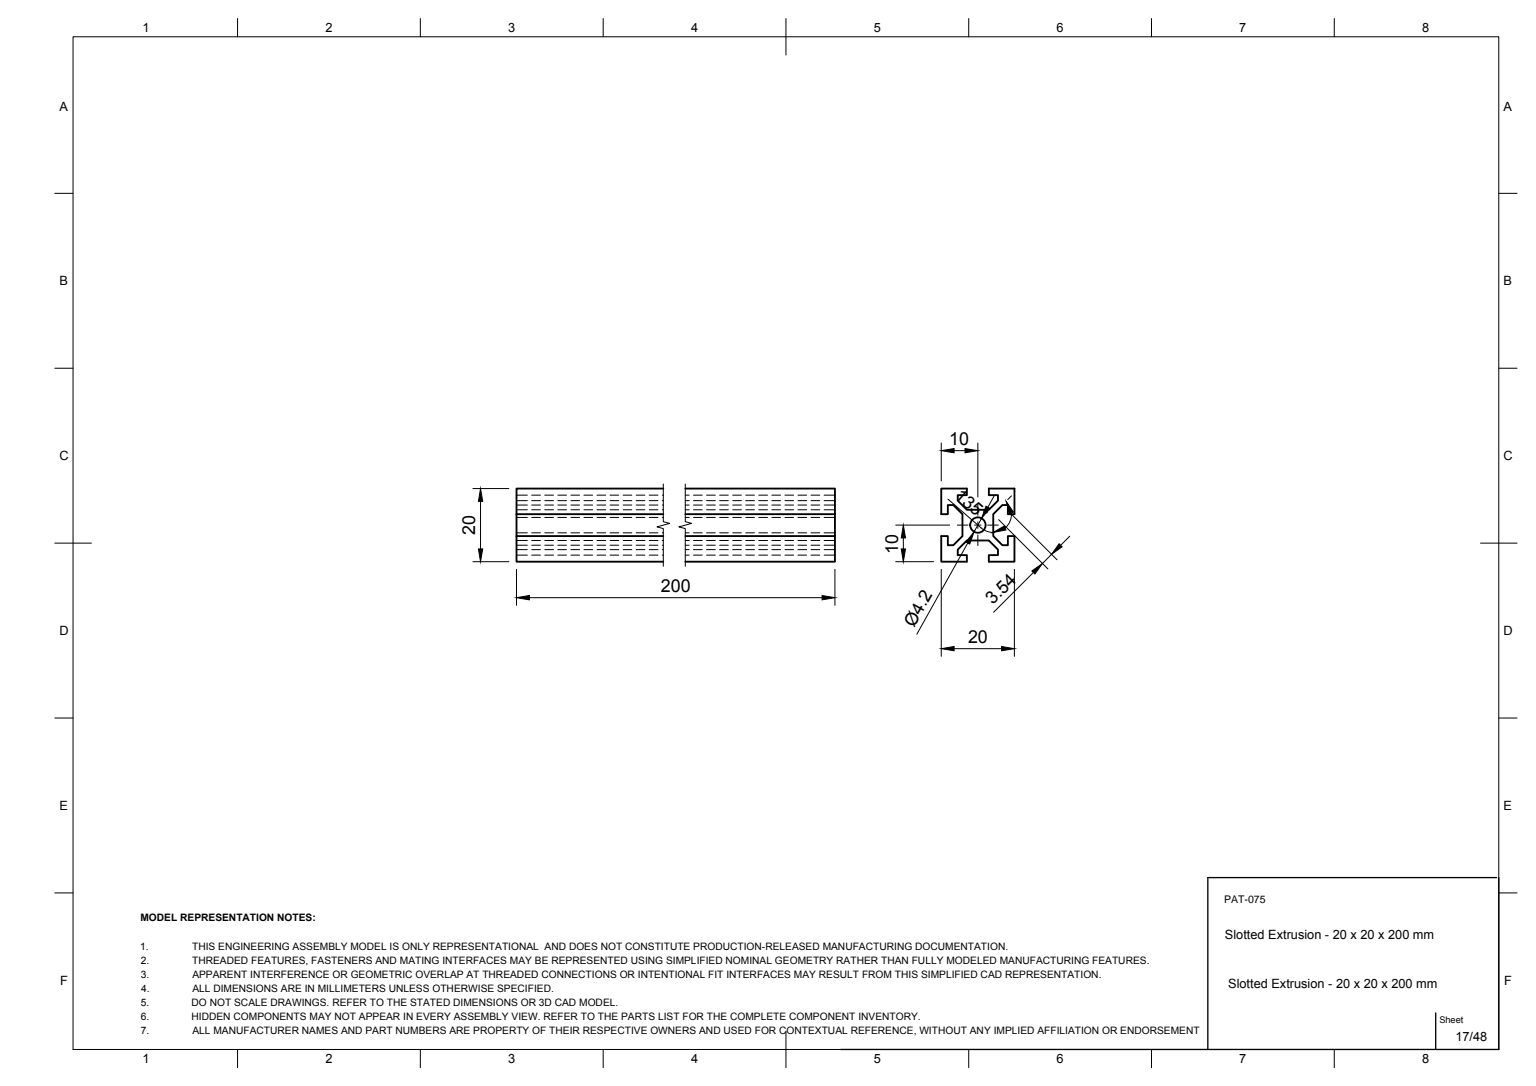
ISO-10303-21;
HEADER;
/* Generated by software containing ST-Developer
 * from STEP Tools, Inc. (www.steptools.com) 
 */

FILE_DESCRIPTION(
/* description */ ('Over-Centre Plunger Toggle Clamp on Slotted Fixture Frame'),
/* implementation_level */ '2;1');

FILE_NAME(
/* name */ 
'Slotted Extrusion - 20 x 20 x 200 mm.step',
/* time_stamp */ '2026-10-28T03:23:24-07:00',
/* author */ (''),
/* organization */ (''),
/* preprocessor_version */ 'ST-DEVELOPER v20.2',
/* originating_system */ 'Autodesk Translation Framework v15.17.0.0',
/* authorisation */ '');

FILE_SCHEMA (('AUTOMOTIVE_DESIGN { 1 0 10303 214 3 1 1 }'));
ENDSEC;

DATA;
#10=MECHANICAL_DESIGN_GEOMETRIC_PRESENTATION_REPRESENTATION('',(#525),#15212);
#441=SHAPE_REPRESENTATION_RELATIONSHIP('SRR','None',#15415,#483);
#483=ADVANCED_BREP_SHAPE_REPRESENTATION('',(#576),#15177);
#525=STYLED_ITEM('',(#15733),#576);
#576=MANIFOLD_SOLID_BREP('Body1',#8257);
#714=FACE_BOUND('',#1871,.T.);
#715=FACE_BOUND('',#1873,.T.);
#866=PLANE('',#9059);
#867=PLANE('',#9060);
#868=PLANE('',#9061);
#869=PLANE('',#9062);
#870=PLANE('',#9063);
#871=PLANE('',#9064);
#872=PLANE('',#9065);
#873=PLANE('',#9066);
#874=PLANE('',#9067);
#875=PLANE('',#9068);
#876=PLANE('',#9069);
#877=PLANE('',#9070);
#878=PLANE('',#9071);
#879=PLANE('',#9072);
#880=PLANE('',#9073);
#881=PLANE('',#9074);
#882=PLANE('',#9075);
#883=PLANE('',#9076);
#884=PLANE('',#9077);
#885=PLANE('',#9078);
#886=PLANE('',#9079);
#887=PLANE('',#9080);
#888=PLANE('',#9081);
#889=PLANE('',#9082);
#890=PLANE('',#9083);
#891=PLANE('',#9084);
#892=PLANE('',#9085);
#893=PLANE('',#9086);
#894=PLANE('',#9087);
#895=PLANE('',#9088);
#896=PLANE('',#9089);
#897=PLANE('',#9090);
#898=PLANE('',#9091);
#899=PLANE('',#9092);
#900=PLANE('',#9093);
#901=PLANE('',#9094);
#902=PLANE('',#9098);
#903=PLANE('',#9099);
#904=PLANE('',#9100);
#905=PLANE('',#9101);
#906=PLANE('',#9102);
#907=PLANE('',#9103);
#908=PLANE('',#9104);
#909=PLANE('',#9105);
#910=PLANE('',#9106);
#911=PLANE('',#9107);
#1236=FACE_OUTER_BOUND('',#1825,.T.);
#1237=FACE_OUTER_BOUND('',#1826,.T.);
#1238=FACE_OUTER_BOUND('',#1827,.T.);
#1239=FACE_OUTER_BOUND('',#1828,.T.);
#1240=FACE_OUTER_BOUND('',#1829,.T.);
#1241=FACE_OUTER_BOUND('',#1830,.T.);
#1242=FACE_OUTER_BOUND('',#1831,.T.);
#1243=FACE_OUTER_BOUND('',#1832,.T.);
#1244=FACE_OUTER_BOUND('',#1833,.T.);
#1245=FACE_OUTER_BOUND('',#1834,.T.);
#1246=FACE_OUTER_BOUND('',#1835,.T.);
#1247=FACE_OUTER_BOUND('',#1836,.T.);
#1248=FACE_OUTER_BOUND('',#1837,.T.);
#1249=FACE_OUTER_BOUND('',#1838,.T.);
#1250=FACE_OUTER_BOUND('',#1839,.T.);
#1251=FACE_OUTER_BOUND('',#1840,.T.);
#1252=FACE_OUTER_BOUND('',#1841,.T.);
#1253=FACE_OUTER_BOUND('',#1842,.T.);
#1254=FACE_OUTER_BOUND('',#1843,.T.);
#1255=FACE_OUTER_BOUND('',#1844,.T.);
#1256=FACE_OUTER_BOUND('',#1845,.T.);
#1257=FACE_OUTER_BOUND('',#1846,.T.);
#1258=FACE_OUTER_BOUND('',#1847,.T.);
#1259=FACE_OUTER_BOUND('',#1848,.T.);
#1260=FACE_OUTER_BOUND('',#1849,.T.);
#1261=FACE_OUTER_BOUND('',#1850,.T.);
#1262=FACE_OUTER_BOUND('',#1851,.T.);
#1263=FACE_OUTER_BOUND('',#1852,.T.);
#1264=FACE_OUTER_BOUND('',#1853,.T.);
#1265=FACE_OUTER_BOUND('',#1854,.T.);
#1266=FACE_OUTER_BOUND('',#1855,.T.);
#1267=FACE_OUTER_BOUND('',#1856,.T.);
#1268=FACE_OUTER_BOUND('',#1857,.T.);
#1269=FACE_OUTER_BOUND('',#1858,.T.);
#1270=FACE_OUTER_BOUND('',#1859,.T.);
#1271=FACE_OUTER_BOUND('',#1860,.T.);
#1272=FACE_OUTER_BOUND('',#1861,.T.);
#1273=FACE_OUTER_BOUND('',#1862,.T.);
#1274=FACE_OUTER_BOUND('',#1863,.T.);
#1275=FACE_OUTER_BOUND('',#1864,.T.);
#1276=FACE_OUTER_BOUND('',#1865,.T.);
#1277=FACE_OUTER_BOUND('',#1866,.T.);
#1278=FACE_OUTER_BOUND('',#1867,.T.);
#1279=FACE_OUTER_BOUND('',#1868,.T.);
#1280=FACE_OUTER_BOUND('',#1869,.T.);
#1281=FACE_OUTER_BOUND('',#1870,.T.);
#1282=FACE_OUTER_BOUND('',#1872,.T.);
#1825=EDGE_LOOP('',(#6205,#6206,#6207,#6208));
#1826=EDGE_LOOP('',(#6209,#6210,#6211,#6212));
#1827=EDGE_LOOP('',(#6213,#6214,#6215,#6216));
#1828=EDGE_LOOP('',(#6217,#6218,#6219,#6220));
#1829=EDGE_LOOP('',(#6221,#6222,#6223,#6224));
#1830=EDGE_LOOP('',(#6225,#6226,#6227,#6228));
#1831=EDGE_LOOP('',(#6229,#6230,#6231,#6232));
#1832=EDGE_LOOP('',(#6233,#6234,#6235,#6236));
#1833=EDGE_LOOP('',(#6237,#6238,#6239,#6240));
#1834=EDGE_LOOP('',(#6241,#6242,#6243,#6244));
#1835=EDGE_LOOP('',(#6245,#6246,#6247,#6248));
#1836=EDGE_LOOP('',(#6249,#6250,#6251,#6252));
#1837=EDGE_LOOP('',(#6253,#6254,#6255,#6256));
#1838=EDGE_LOOP('',(#6257,#6258,#6259,#6260));
#1839=EDGE_LOOP('',(#6261,#6262,#6263,#6264));
#1840=EDGE_LOOP('',(#6265,#6266,#6267,#6268));
#1841=EDGE_LOOP('',(#6269,#6270,#6271,#6272));
#1842=EDGE_LOOP('',(#6273,#6274,#6275,#6276));
#1843=EDGE_LOOP('',(#6277,#6278,#6279,#6280));
#1844=EDGE_LOOP('',(#6281,#6282,#6283,#6284));
#1845=EDGE_LOOP('',(#6285,#6286,#6287,#6288));
#1846=EDGE_LOOP('',(#6289,#6290,#6291,#6292));
#1847=EDGE_LOOP('',(#6293,#6294,#6295,#6296));
#1848=EDGE_LOOP('',(#6297,#6298,#6299,#6300));
#1849=EDGE_LOOP('',(#6301,#6302,#6303,#6304));
#1850=EDGE_LOOP('',(#6305,#6306,#6307,#6308));
#1851=EDGE_LOOP('',(#6309,#6310,#6311,#6312));
#1852=EDGE_LOOP('',(#6313,#6314,#6315,#6316));
#1853=EDGE_LOOP('',(#6317,#6318,#6319,#6320));
#1854=EDGE_LOOP('',(#6321,#6322,#6323,#6324));
#1855=EDGE_LOOP('',(#6325,#6326,#6327,#6328));
#1856=EDGE_LOOP('',(#6329,#6330,#6331,#6332));
#1857=EDGE_LOOP('',(#6333,#6334,#6335,#6336));
#1858=EDGE_LOOP('',(#6337,#6338,#6339,#6340));
#1859=EDGE_LOOP('',(#6341,#6342,#6343,#6344));
#1860=EDGE_LOOP('',(#6345,#6346,#6347,#6348));
#1861=EDGE_LOOP('',(#6349,#6350,#6351,#6352));
#1862=EDGE_LOOP('',(#6353,#6354,#6355,#6356));
#1863=EDGE_LOOP('',(#6357,#6358,#6359,#6360));
#1864=EDGE_LOOP('',(#6361,#6362,#6363,#6364));
#1865=EDGE_LOOP('',(#6365,#6366,#6367,#6368));
#1866=EDGE_LOOP('',(#6369,#6370,#6371,#6372));
#1867=EDGE_LOOP('',(#6373,#6374,#6375,#6376));
#1868=EDGE_LOOP('',(#6377,#6378,#6379,#6380));
#1869=EDGE_LOOP('',(#6381,#6382,#6383,#6384));
#1870=EDGE_LOOP('',(#6385,#6386,#6387,#6388,#6389,#6390,#6391,#6392,#6393,
#6394,#6395,#6396,#6397,#6398,#6399,#6400,#6401,#6402,#6403,#6404,#6405,
#6406,#6407,#6408,#6409,#6410,#6411,#6412,#6413,#6414,#6415,#6416,#6417,
#6418,#6419,#6420,#6421,#6422,#6423,#6424,#6425,#6426,#6427,#6428));
#1871=EDGE_LOOP('',(#6429));
#1872=EDGE_LOOP('',(#6430,#6431,#6432,#6433,#6434,#6435,#6436,#6437,#6438,
#6439,#6440,#6441,#6442,#6443,#6444,#6445,#6446,#6447,#6448,#6449,#6450,
#6451,#6452,#6453,#6454,#6455,#6456,#6457,#6458,#6459,#6460,#6461,#6462,
#6463,#6464,#6465,#6466,#6467,#6468,#6469,#6470,#6471,#6472,#6473));
#1873=EDGE_LOOP('',(#6474));
#2417=LINE('',#13063,#3047);
#2418=LINE('',#13065,#3048);
#2419=LINE('',#13067,#3049);
#2420=LINE('',#13068,#3050);
#2421=LINE('',#13071,#3051);
#2422=LINE('',#13073,#3052);
#2423=LINE('',#13074,#3053);
#2424=LINE('',#13077,#3054);
#2425=LINE('',#13079,#3055);
#2426=LINE('',#13080,#3056);
#2427=LINE('',#13083,#3057);
#2428=LINE('',#13085,#3058);
#2429=LINE('',#13086,#3059);
#2430=LINE('',#13089,#3060);
#2431=LINE('',#13091,#3061);
#2432=LINE('',#13092,#3062);
#2433=LINE('',#13095,#3063);
#2434=LINE('',#13097,#3064);
#2435=LINE('',#13098,#3065);
#2436=LINE('',#13101,#3066);
#2437=LINE('',#13103,#3067);
#2438=LINE('',#13104,#3068);
#2439=LINE('',#13107,#3069);
#2440=LINE('',#13109,#3070);
#2441=LINE('',#13110,#3071);
#2442=LINE('',#13113,#3072);
#2443=LINE('',#13115,#3073);
#2444=LINE('',#13116,#3074);
#2445=LINE('',#13120,#3075);
#2446=LINE('',#13122,#3076);
#2447=LINE('',#13124,#3077);
#2448=LINE('',#13125,#3078);
#2449=LINE('',#13128,#3079);
#2450=LINE('',#13130,#3080);
#2451=LINE('',#13131,#3081);
#2452=LINE('',#13134,#3082);
#2453=LINE('',#13136,#3083);
#2454=LINE('',#13137,#3084);
#2455=LINE('',#13140,#3085);
#2456=LINE('',#13142,#3086);
#2457=LINE('',#13143,#3087);
#2458=LINE('',#13146,#3088);
#2459=LINE('',#13148,#3089);
#2460=LINE('',#13149,#3090);
#2461=LINE('',#13152,#3091);
#2462=LINE('',#13154,#3092);
#2463=LINE('',#13155,#3093);
#2464=LINE('',#13158,#3094);
#2465=LINE('',#13160,#3095);
#2466=LINE('',#13161,#3096);
#2467=LINE('',#13164,#3097);
#2468=LINE('',#13166,#3098);
#2469=LINE('',#13167,#3099);
#2470=LINE('',#13170,#3100);
#2471=LINE('',#13172,#3101);
#2472=LINE('',#13173,#3102);
#2473=LINE('',#13177,#3103);
#2474=LINE('',#13179,#3104);
#2475=LINE('',#13181,#3105);
#2476=LINE('',#13182,#3106);
#2477=LINE('',#13185,#3107);
#2478=LINE('',#13187,#3108);
#2479=LINE('',#13188,#3109);
#2480=LINE('',#13191,#3110);
#2481=LINE('',#13193,#3111);
#2482=LINE('',#13194,#3112);
#2483=LINE('',#13197,#3113);
#2484=LINE('',#13199,#3114);
#2485=LINE('',#13200,#3115);
#2486=LINE('',#13203,#3116);
#2487=LINE('',#13205,#3117);
#2488=LINE('',#13206,#3118);
#2489=LINE('',#13209,#3119);
#2490=LINE('',#13211,#3120);
#2491=LINE('',#13212,#3121);
#2492=LINE('',#13215,#3122);
#2493=LINE('',#13217,#3123);
#2494=LINE('',#13218,#3124);
#2495=LINE('',#13221,#3125);
#2496=LINE('',#13223,#3126);
#2497=LINE('',#13224,#3127);
#2498=LINE('',#13227,#3128);
#2499=LINE('',#13229,#3129);
#2500=LINE('',#13230,#3130);
#2501=LINE('',#13234,#3131);
#2502=LINE('',#13236,#3132);
#2503=LINE('',#13238,#3133);
#2504=LINE('',#13239,#3134);
#2505=LINE('',#13242,#3135);
#2506=LINE('',#13244,#3136);
#2507=LINE('',#13245,#3137);
#2508=LINE('',#13248,#3138);
#2509=LINE('',#13250,#3139);
#2510=LINE('',#13251,#3140);
#2511=LINE('',#13254,#3141);
#2512=LINE('',#13256,#3142);
#2513=LINE('',#13257,#3143);
#2514=LINE('',#13260,#3144);
#2515=LINE('',#13262,#3145);
#2516=LINE('',#13263,#3146);
#2517=LINE('',#13266,#3147);
#2518=LINE('',#13268,#3148);
#2519=LINE('',#13269,#3149);
#2520=LINE('',#13272,#3150);
#2521=LINE('',#13274,#3151);
#2522=LINE('',#13275,#3152);
#2523=LINE('',#13278,#3153);
#2524=LINE('',#13280,#3154);
#2525=LINE('',#13281,#3155);
#2526=LINE('',#13284,#3156);
#2527=LINE('',#13286,#3157);
#2528=LINE('',#13287,#3158);
#2529=LINE('',#13292,#3159);
#2530=LINE('',#13296,#3160);
#2531=LINE('',#13298,#3161);
#2532=LINE('',#13299,#3162);
#2533=LINE('',#13302,#3163);
#2534=LINE('',#13304,#3164);
#2535=LINE('',#13305,#3165);
#2536=LINE('',#13307,#3166);
#2537=LINE('',#13308,#3167);
#2538=LINE('',#13311,#3168);
#2539=LINE('',#13313,#3169);
#2540=LINE('',#13314,#3170);
#2541=LINE('',#13316,#3171);
#2542=LINE('',#13317,#3172);
#2543=LINE('',#13320,#3173);
#2544=LINE('',#13322,#3174);
#2545=LINE('',#13323,#3175);
#2546=LINE('',#13325,#3176);
#2547=LINE('',#13326,#3177);
#2548=LINE('',#13328,#3178);
#2549=LINE('',#13329,#3179);
#3047=VECTOR('',#10534,1.);
#3048=VECTOR('',#10535,1.);
#3049=VECTOR('',#10536,1.);
#3050=VECTOR('',#10537,1.);
#3051=VECTOR('',#10540,1.);
#3052=VECTOR('',#10541,1.);
#3053=VECTOR('',#10542,1.);
#3054=VECTOR('',#10545,1.);
#3055=VECTOR('',#10546,1.);
#3056=VECTOR('',#10547,1.);
#3057=VECTOR('',#10550,1.);
#3058=VECTOR('',#10551,1.);
#3059=VECTOR('',#10552,1.);
#3060=VECTOR('',#10555,1.);
#3061=VECTOR('',#10556,1.);
#3062=VECTOR('',#10557,1.);
#3063=VECTOR('',#10560,1.);
#3064=VECTOR('',#10561,1.);
#3065=VECTOR('',#10562,1.);
#3066=VECTOR('',#10565,1.);
#3067=VECTOR('',#10566,1.);
#3068=VECTOR('',#10567,1.);
#3069=VECTOR('',#10570,1.);
#3070=VECTOR('',#10571,1.);
#3071=VECTOR('',#10572,1.);
#3072=VECTOR('',#10575,1.);
#3073=VECTOR('',#10576,1.);
#3074=VECTOR('',#10577,1.);
#3075=VECTOR('',#10580,1.);
#3076=VECTOR('',#10581,1.);
#3077=VECTOR('',#10582,1.);
#3078=VECTOR('',#10583,1.);
#3079=VECTOR('',#10586,1.);
#3080=VECTOR('',#10587,1.);
#3081=VECTOR('',#10588,1.);
#3082=VECTOR('',#10591,1.);
#3083=VECTOR('',#10592,1.);
#3084=VECTOR('',#10593,1.);
#3085=VECTOR('',#10596,1.);
#3086=VECTOR('',#10597,1.);
#3087=VECTOR('',#10598,1.);
#3088=VECTOR('',#10601,1.);
#3089=VECTOR('',#10602,1.);
#3090=VECTOR('',#10603,1.);
#3091=VECTOR('',#10606,1.);
#3092=VECTOR('',#10607,1.);
#3093=VECTOR('',#10608,1.);
#3094=VECTOR('',#10611,1.);
#3095=VECTOR('',#10612,1.);
#3096=VECTOR('',#10613,1.);
#3097=VECTOR('',#10616,1.);
#3098=VECTOR('',#10617,1.);
#3099=VECTOR('',#10618,1.);
#3100=VECTOR('',#10621,1.);
#3101=VECTOR('',#10622,1.);
#3102=VECTOR('',#10623,1.);
#3103=VECTOR('',#10626,1.);
#3104=VECTOR('',#10627,1.);
#3105=VECTOR('',#10628,1.);
#3106=VECTOR('',#10629,1.);
#3107=VECTOR('',#10632,1.);
#3108=VECTOR('',#10633,1.);
#3109=VECTOR('',#10634,1.);
#3110=VECTOR('',#10637,1.);
#3111=VECTOR('',#10638,1.);
#3112=VECTOR('',#10639,1.);
#3113=VECTOR('',#10642,1.);
#3114=VECTOR('',#10643,1.);
#3115=VECTOR('',#10644,1.);
#3116=VECTOR('',#10647,1.);
#3117=VECTOR('',#10648,1.);
#3118=VECTOR('',#10649,1.);
#3119=VECTOR('',#10652,1.);
#3120=VECTOR('',#10653,1.);
#3121=VECTOR('',#10654,1.);
#3122=VECTOR('',#10657,1.);
#3123=VECTOR('',#10658,1.);
#3124=VECTOR('',#10659,1.);
#3125=VECTOR('',#10662,1.);
#3126=VECTOR('',#10663,1.);
#3127=VECTOR('',#10664,1.);
#3128=VECTOR('',#10667,1.);
#3129=VECTOR('',#10668,1.);
#3130=VECTOR('',#10669,1.);
#3131=VECTOR('',#10672,1.);
#3132=VECTOR('',#10673,1.);
#3133=VECTOR('',#10674,1.);
#3134=VECTOR('',#10675,1.);
#3135=VECTOR('',#10678,1.);
#3136=VECTOR('',#10679,1.);
#3137=VECTOR('',#10680,1.);
#3138=VECTOR('',#10683,1.);
#3139=VECTOR('',#10684,1.);
#3140=VECTOR('',#10685,1.);
#3141=VECTOR('',#10688,1.);
#3142=VECTOR('',#10689,1.);
#3143=VECTOR('',#10690,1.);
#3144=VECTOR('',#10693,1.);
#3145=VECTOR('',#10694,1.);
#3146=VECTOR('',#10695,1.);
#3147=VECTOR('',#10698,1.);
#3148=VECTOR('',#10699,1.);
#3149=VECTOR('',#10700,1.);
#3150=VECTOR('',#10703,1.);
#3151=VECTOR('',#10704,1.);
#3152=VECTOR('',#10705,1.);
#3153=VECTOR('',#10708,1.);
#3154=VECTOR('',#10709,1.);
#3155=VECTOR('',#10710,1.);
#3156=VECTOR('',#10713,1.);
#3157=VECTOR('',#10714,1.);
#3158=VECTOR('',#10715,1.);
#3159=VECTOR('',#10720,0.21);
#3160=VECTOR('',#10725,1.);
#3161=VECTOR('',#10726,1.);
#3162=VECTOR('',#10727,1.);
#3163=VECTOR('',#10730,1.);
#3164=VECTOR('',#10731,1.);
#3165=VECTOR('',#10732,1.);
#3166=VECTOR('',#10735,1.);
#3167=VECTOR('',#10736,1.);
#3168=VECTOR('',#10739,1.);
#3169=VECTOR('',#10740,1.);
#3170=VECTOR('',#10741,1.);
#3171=VECTOR('',#10744,1.);
#3172=VECTOR('',#10745,1.);
#3173=VECTOR('',#10748,1.);
#3174=VECTOR('',#10749,1.);
#3175=VECTOR('',#10750,1.);
#3176=VECTOR('',#10753,1.);
#3177=VECTOR('',#10754,1.);
#3178=VECTOR('',#10757,1.);
#3179=VECTOR('',#10758,1.);
#3623=CIRCLE('',#9096,0.21);
#3624=CIRCLE('',#9097,0.21);
#4071=VERTEX_POINT('',#13061);
#4072=VERTEX_POINT('',#13062);
#4073=VERTEX_POINT('',#13064);
#4074=VERTEX_POINT('',#13066);
#4075=VERTEX_POINT('',#13070);
#4076=VERTEX_POINT('',#13072);
#4077=VERTEX_POINT('',#13076);
#4078=VERTEX_POINT('',#13078);
#4079=VERTEX_POINT('',#13082);
#4080=VERTEX_POINT('',#13084);
#4081=VERTEX_POINT('',#13088);
#4082=VERTEX_POINT('',#13090);
#4083=VERTEX_POINT('',#13094);
#4084=VERTEX_POINT('',#13096);
#4085=VERTEX_POINT('',#13100);
#4086=VERTEX_POINT('',#13102);
#4087=VERTEX_POINT('',#13106);
#4088=VERTEX_POINT('',#13108);
#4089=VERTEX_POINT('',#13112);
#4090=VERTEX_POINT('',#13114);
#4091=VERTEX_POINT('',#13118);
#4092=VERTEX_POINT('',#13119);
#4093=VERTEX_POINT('',#13121);
#4094=VERTEX_POINT('',#13123);
#4095=VERTEX_POINT('',#13127);
#4096=VERTEX_POINT('',#13129);
#4097=VERTEX_POINT('',#13133);
#4098=VERTEX_POINT('',#13135);
#4099=VERTEX_POINT('',#13139);
#4100=VERTEX_POINT('',#13141);
#4101=VERTEX_POINT('',#13145);
#4102=VERTEX_POINT('',#13147);
#4103=VERTEX_POINT('',#13151);
#4104=VERTEX_POINT('',#13153);
#4105=VERTEX_POINT('',#13157);
#4106=VERTEX_POINT('',#13159);
#4107=VERTEX_POINT('',#13163);
#4108=VERTEX_POINT('',#13165);
#4109=VERTEX_POINT('',#13169);
#4110=VERTEX_POINT('',#13171);
#4111=VERTEX_POINT('',#13175);
#4112=VERTEX_POINT('',#13176);
#4113=VERTEX_POINT('',#13178);
#4114=VERTEX_POINT('',#13180);
#4115=VERTEX_POINT('',#13184);
#4116=VERTEX_POINT('',#13186);
#4117=VERTEX_POINT('',#13190);
#4118=VERTEX_POINT('',#13192);
#4119=VERTEX_POINT('',#13196);
#4120=VERTEX_POINT('',#13198);
#4121=VERTEX_POINT('',#13202);
#4122=VERTEX_POINT('',#13204);
#4123=VERTEX_POINT('',#13208);
#4124=VERTEX_POINT('',#13210);
#4125=VERTEX_POINT('',#13214);
#4126=VERTEX_POINT('',#13216);
#4127=VERTEX_POINT('',#13220);
#4128=VERTEX_POINT('',#13222);
#4129=VERTEX_POINT('',#13226);
#4130=VERTEX_POINT('',#13228);
#4131=VERTEX_POINT('',#13232);
#4132=VERTEX_POINT('',#13233);
#4133=VERTEX_POINT('',#13235);
#4134=VERTEX_POINT('',#13237);
#4135=VERTEX_POINT('',#13241);
#4136=VERTEX_POINT('',#13243);
#4137=VERTEX_POINT('',#13247);
#4138=VERTEX_POINT('',#13249);
#4139=VERTEX_POINT('',#13253);
#4140=VERTEX_POINT('',#13255);
#4141=VERTEX_POINT('',#13259);
#4142=VERTEX_POINT('',#13261);
#4143=VERTEX_POINT('',#13265);
#4144=VERTEX_POINT('',#13267);
#4145=VERTEX_POINT('',#13271);
#4146=VERTEX_POINT('',#13273);
#4147=VERTEX_POINT('',#13277);
#4148=VERTEX_POINT('',#13279);
#4149=VERTEX_POINT('',#13283);
#4150=VERTEX_POINT('',#13285);
#4151=VERTEX_POINT('',#13289);
#4152=VERTEX_POINT('',#13291);
#4153=VERTEX_POINT('',#13295);
#4154=VERTEX_POINT('',#13297);
#4155=VERTEX_POINT('',#13301);
#4156=VERTEX_POINT('',#13303);
#4157=VERTEX_POINT('',#13310);
#4158=VERTEX_POINT('',#13312);
#4159=VERTEX_POINT('',#13319);
#4160=VERTEX_POINT('',#13321);
#4863=EDGE_CURVE('',#4071,#4072,#2417,.T.);
#4864=EDGE_CURVE('',#4071,#4073,#2418,.T.);
#4865=EDGE_CURVE('',#4074,#4073,#2419,.T.);
#4866=EDGE_CURVE('',#4072,#4074,#2420,.T.);
#4867=EDGE_CURVE('',#4075,#4071,#2421,.T.);
#4868=EDGE_CURVE('',#4075,#4076,#2422,.T.);
#4869=EDGE_CURVE('',#4073,#4076,#2423,.T.);
#4870=EDGE_CURVE('',#4077,#4075,#2424,.T.);
#4871=EDGE_CURVE('',#4077,#4078,#2425,.T.);
#4872=EDGE_CURVE('',#4076,#4078,#2426,.T.);
#4873=EDGE_CURVE('',#4079,#4077,#2427,.T.);
#4874=EDGE_CURVE('',#4079,#4080,#2428,.T.);
#4875=EDGE_CURVE('',#4078,#4080,#2429,.T.);
#4876=EDGE_CURVE('',#4081,#4079,#2430,.T.);
#4877=EDGE_CURVE('',#4081,#4082,#2431,.T.);
#4878=EDGE_CURVE('',#4080,#4082,#2432,.T.);
#4879=EDGE_CURVE('',#4083,#4081,#2433,.T.);
#4880=EDGE_CURVE('',#4083,#4084,#2434,.T.);
#4881=EDGE_CURVE('',#4082,#4084,#2435,.T.);
#4882=EDGE_CURVE('',#4085,#4083,#2436,.T.);
#4883=EDGE_CURVE('',#4085,#4086,#2437,.T.);
#4884=EDGE_CURVE('',#4084,#4086,#2438,.T.);
#4885=EDGE_CURVE('',#4087,#4085,#2439,.T.);
#4886=EDGE_CURVE('',#4087,#4088,#2440,.T.);
#4887=EDGE_CURVE('',#4086,#4088,#2441,.T.);
#4888=EDGE_CURVE('',#4089,#4087,#2442,.T.);
#4889=EDGE_CURVE('',#4090,#4089,#2443,.T.);
#4890=EDGE_CURVE('',#4088,#4090,#2444,.T.);
#4891=EDGE_CURVE('',#4091,#4092,#2445,.T.);
#4892=EDGE_CURVE('',#4091,#4093,#2446,.T.);
#4893=EDGE_CURVE('',#4094,#4093,#2447,.T.);
#4894=EDGE_CURVE('',#4092,#4094,#2448,.T.);
#4895=EDGE_CURVE('',#4095,#4091,#2449,.T.);
#4896=EDGE_CURVE('',#4095,#4096,#2450,.T.);
#4897=EDGE_CURVE('',#4093,#4096,#2451,.T.);
#4898=EDGE_CURVE('',#4097,#4095,#2452,.T.);
#4899=EDGE_CURVE('',#4097,#4098,#2453,.T.);
#4900=EDGE_CURVE('',#4096,#4098,#2454,.T.);
#4901=EDGE_CURVE('',#4099,#4097,#2455,.T.);
#4902=EDGE_CURVE('',#4099,#4100,#2456,.T.);
#4903=EDGE_CURVE('',#4098,#4100,#2457,.T.);
#4904=EDGE_CURVE('',#4101,#4099,#2458,.T.);
#4905=EDGE_CURVE('',#4101,#4102,#2459,.T.);
#4906=EDGE_CURVE('',#4100,#4102,#2460,.T.);
#4907=EDGE_CURVE('',#4103,#4101,#2461,.T.);
#4908=EDGE_CURVE('',#4103,#4104,#2462,.T.);
#4909=EDGE_CURVE('',#4102,#4104,#2463,.T.);
#4910=EDGE_CURVE('',#4105,#4103,#2464,.T.);
#4911=EDGE_CURVE('',#4105,#4106,#2465,.T.);
#4912=EDGE_CURVE('',#4104,#4106,#2466,.T.);
#4913=EDGE_CURVE('',#4107,#4105,#2467,.T.);
#4914=EDGE_CURVE('',#4107,#4108,#2468,.T.);
#4915=EDGE_CURVE('',#4106,#4108,#2469,.T.);
#4916=EDGE_CURVE('',#4109,#4107,#2470,.T.);
#4917=EDGE_CURVE('',#4110,#4109,#2471,.T.);
#4918=EDGE_CURVE('',#4108,#4110,#2472,.T.);
#4919=EDGE_CURVE('',#4111,#4112,#2473,.T.);
#4920=EDGE_CURVE('',#4111,#4113,#2474,.T.);
#4921=EDGE_CURVE('',#4114,#4113,#2475,.T.);
#4922=EDGE_CURVE('',#4112,#4114,#2476,.T.);
#4923=EDGE_CURVE('',#4115,#4111,#2477,.T.);
#4924=EDGE_CURVE('',#4115,#4116,#2478,.T.);
#4925=EDGE_CURVE('',#4113,#4116,#2479,.T.);
#4926=EDGE_CURVE('',#4117,#4115,#2480,.T.);
#4927=EDGE_CURVE('',#4117,#4118,#2481,.T.);
#4928=EDGE_CURVE('',#4116,#4118,#2482,.T.);
#4929=EDGE_CURVE('',#4119,#4117,#2483,.T.);
#4930=EDGE_CURVE('',#4119,#4120,#2484,.T.);
#4931=EDGE_CURVE('',#4118,#4120,#2485,.T.);
#4932=EDGE_CURVE('',#4121,#4119,#2486,.T.);
#4933=EDGE_CURVE('',#4121,#4122,#2487,.T.);
#4934=EDGE_CURVE('',#4120,#4122,#2488,.T.);
#4935=EDGE_CURVE('',#4123,#4121,#2489,.T.);
#4936=EDGE_CURVE('',#4123,#4124,#2490,.T.);
#4937=EDGE_CURVE('',#4122,#4124,#2491,.T.);
#4938=EDGE_CURVE('',#4125,#4123,#2492,.T.);
#4939=EDGE_CURVE('',#4125,#4126,#2493,.T.);
#4940=EDGE_CURVE('',#4124,#4126,#2494,.T.);
#4941=EDGE_CURVE('',#4127,#4125,#2495,.T.);
#4942=EDGE_CURVE('',#4127,#4128,#2496,.T.);
#4943=EDGE_CURVE('',#4126,#4128,#2497,.T.);
#4944=EDGE_CURVE('',#4129,#4127,#2498,.T.);
#4945=EDGE_CURVE('',#4130,#4129,#2499,.T.);
#4946=EDGE_CURVE('',#4128,#4130,#2500,.T.);
#4947=EDGE_CURVE('',#4131,#4132,#2501,.T.);
#4948=EDGE_CURVE('',#4131,#4133,#2502,.T.);
#4949=EDGE_CURVE('',#4134,#4133,#2503,.T.);
#4950=EDGE_CURVE('',#4132,#4134,#2504,.T.);
#4951=EDGE_CURVE('',#4135,#4131,#2505,.T.);
#4952=EDGE_CURVE('',#4135,#4136,#2506,.T.);
#4953=EDGE_CURVE('',#4133,#4136,#2507,.T.);
#4954=EDGE_CURVE('',#4137,#4135,#2508,.T.);
#4955=EDGE_CURVE('',#4137,#4138,#2509,.T.);
#4956=EDGE_CURVE('',#4136,#4138,#2510,.T.);
#4957=EDGE_CURVE('',#4139,#4137,#2511,.T.);
#4958=EDGE_CURVE('',#4139,#4140,#2512,.T.);
#4959=EDGE_CURVE('',#4138,#4140,#2513,.T.);
#4960=EDGE_CURVE('',#4141,#4139,#2514,.T.);
#4961=EDGE_CURVE('',#4141,#4142,#2515,.T.);
#4962=EDGE_CURVE('',#4140,#4142,#2516,.T.);
#4963=EDGE_CURVE('',#4143,#4141,#2517,.T.);
#4964=EDGE_CURVE('',#4143,#4144,#2518,.T.);
#4965=EDGE_CURVE('',#4142,#4144,#2519,.T.);
#4966=EDGE_CURVE('',#4145,#4143,#2520,.T.);
#4967=EDGE_CURVE('',#4145,#4146,#2521,.T.);
#4968=EDGE_CURVE('',#4144,#4146,#2522,.T.);
#4969=EDGE_CURVE('',#4147,#4145,#2523,.T.);
#4970=EDGE_CURVE('',#4147,#4148,#2524,.T.);
#4971=EDGE_CURVE('',#4146,#4148,#2525,.T.);
#4972=EDGE_CURVE('',#4149,#4147,#2526,.T.);
#4973=EDGE_CURVE('',#4150,#4149,#2527,.T.);
#4974=EDGE_CURVE('',#4148,#4150,#2528,.T.);
#4975=EDGE_CURVE('',#4151,#4151,#3623,.T.);
#4976=EDGE_CURVE('',#4151,#4152,#2529,.T.);
#4977=EDGE_CURVE('',#4152,#4152,#3624,.T.);
#4978=EDGE_CURVE('',#4089,#4153,#2530,.T.);
#4979=EDGE_CURVE('',#4153,#4154,#2531,.T.);
#4980=EDGE_CURVE('',#4090,#4154,#2532,.T.);
#4981=EDGE_CURVE('',#4155,#4074,#2533,.T.);
#4982=EDGE_CURVE('',#4156,#4155,#2534,.T.);
#4983=EDGE_CURVE('',#4156,#4072,#2535,.T.);
#4984=EDGE_CURVE('',#4109,#4156,#2536,.T.);
#4985=EDGE_CURVE('',#4110,#4155,#2537,.T.);
#4986=EDGE_CURVE('',#4157,#4094,#2538,.T.);
#4987=EDGE_CURVE('',#4158,#4157,#2539,.T.);
#4988=EDGE_CURVE('',#4158,#4092,#2540,.T.);
#4989=EDGE_CURVE('',#4129,#4158,#2541,.T.);
#4990=EDGE_CURVE('',#4130,#4157,#2542,.T.);
#4991=EDGE_CURVE('',#4159,#4114,#2543,.T.);
#4992=EDGE_CURVE('',#4160,#4159,#2544,.T.);
#4993=EDGE_CURVE('',#4160,#4112,#2545,.T.);
#4994=EDGE_CURVE('',#4149,#4160,#2546,.T.);
#4995=EDGE_CURVE('',#4150,#4159,#2547,.T.);
#4996=EDGE_CURVE('',#4154,#4134,#2548,.T.);
#4997=EDGE_CURVE('',#4153,#4132,#2549,.T.);
#6205=ORIENTED_EDGE('',*,*,#4863,.F.);
#6206=ORIENTED_EDGE('',*,*,#4864,.T.);
#6207=ORIENTED_EDGE('',*,*,#4865,.F.);
#6208=ORIENTED_EDGE('',*,*,#4866,.F.);
#6209=ORIENTED_EDGE('',*,*,#4867,.F.);
#6210=ORIENTED_EDGE('',*,*,#4868,.T.);
#6211=ORIENTED_EDGE('',*,*,#4869,.F.);
#6212=ORIENTED_EDGE('',*,*,#4864,.F.);
#6213=ORIENTED_EDGE('',*,*,#4870,.F.);
#6214=ORIENTED_EDGE('',*,*,#4871,.T.);
#6215=ORIENTED_EDGE('',*,*,#4872,.F.);
#6216=ORIENTED_EDGE('',*,*,#4868,.F.);
#6217=ORIENTED_EDGE('',*,*,#4873,.F.);
#6218=ORIENTED_EDGE('',*,*,#4874,.T.);
#6219=ORIENTED_EDGE('',*,*,#4875,.F.);
#6220=ORIENTED_EDGE('',*,*,#4871,.F.);
#6221=ORIENTED_EDGE('',*,*,#4876,.F.);
#6222=ORIENTED_EDGE('',*,*,#4877,.T.);
#6223=ORIENTED_EDGE('',*,*,#4878,.F.);
#6224=ORIENTED_EDGE('',*,*,#4874,.F.);
#6225=ORIENTED_EDGE('',*,*,#4879,.F.);
#6226=ORIENTED_EDGE('',*,*,#4880,.T.);
#6227=ORIENTED_EDGE('',*,*,#4881,.F.);
#6228=ORIENTED_EDGE('',*,*,#4877,.F.);
#6229=ORIENTED_EDGE('',*,*,#4882,.F.);
#6230=ORIENTED_EDGE('',*,*,#4883,.T.);
#6231=ORIENTED_EDGE('',*,*,#4884,.F.);
#6232=ORIENTED_EDGE('',*,*,#4880,.F.);
#6233=ORIENTED_EDGE('',*,*,#4885,.F.);
#6234=ORIENTED_EDGE('',*,*,#4886,.T.);
#6235=ORIENTED_EDGE('',*,*,#4887,.F.);
#6236=ORIENTED_EDGE('',*,*,#4883,.F.);
#6237=ORIENTED_EDGE('',*,*,#4888,.F.);
#6238=ORIENTED_EDGE('',*,*,#4889,.F.);
#6239=ORIENTED_EDGE('',*,*,#4890,.F.);
#6240=ORIENTED_EDGE('',*,*,#4886,.F.);
#6241=ORIENTED_EDGE('',*,*,#4891,.F.);
#6242=ORIENTED_EDGE('',*,*,#4892,.T.);
#6243=ORIENTED_EDGE('',*,*,#4893,.F.);
#6244=ORIENTED_EDGE('',*,*,#4894,.F.);
#6245=ORIENTED_EDGE('',*,*,#4895,.F.);
#6246=ORIENTED_EDGE('',*,*,#4896,.T.);
#6247=ORIENTED_EDGE('',*,*,#4897,.F.);
#6248=ORIENTED_EDGE('',*,*,#4892,.F.);
#6249=ORIENTED_EDGE('',*,*,#4898,.F.);
#6250=ORIENTED_EDGE('',*,*,#4899,.T.);
#6251=ORIENTED_EDGE('',*,*,#4900,.F.);
#6252=ORIENTED_EDGE('',*,*,#4896,.F.);
#6253=ORIENTED_EDGE('',*,*,#4901,.F.);
#6254=ORIENTED_EDGE('',*,*,#4902,.T.);
#6255=ORIENTED_EDGE('',*,*,#4903,.F.);
#6256=ORIENTED_EDGE('',*,*,#4899,.F.);
#6257=ORIENTED_EDGE('',*,*,#4904,.F.);
#6258=ORIENTED_EDGE('',*,*,#4905,.T.);
#6259=ORIENTED_EDGE('',*,*,#4906,.F.);
#6260=ORIENTED_EDGE('',*,*,#4902,.F.);
#6261=ORIENTED_EDGE('',*,*,#4907,.F.);
#6262=ORIENTED_EDGE('',*,*,#4908,.T.);
#6263=ORIENTED_EDGE('',*,*,#4909,.F.);
#6264=ORIENTED_EDGE('',*,*,#4905,.F.);
#6265=ORIENTED_EDGE('',*,*,#4910,.F.);
#6266=ORIENTED_EDGE('',*,*,#4911,.T.);
#6267=ORIENTED_EDGE('',*,*,#4912,.F.);
#6268=ORIENTED_EDGE('',*,*,#4908,.F.);
#6269=ORIENTED_EDGE('',*,*,#4913,.F.);
#6270=ORIENTED_EDGE('',*,*,#4914,.T.);
#6271=ORIENTED_EDGE('',*,*,#4915,.F.);
#6272=ORIENTED_EDGE('',*,*,#4911,.F.);
#6273=ORIENTED_EDGE('',*,*,#4916,.F.);
#6274=ORIENTED_EDGE('',*,*,#4917,.F.);
#6275=ORIENTED_EDGE('',*,*,#4918,.F.);
#6276=ORIENTED_EDGE('',*,*,#4914,.F.);
#6277=ORIENTED_EDGE('',*,*,#4919,.F.);
#6278=ORIENTED_EDGE('',*,*,#4920,.T.);
#6279=ORIENTED_EDGE('',*,*,#4921,.F.);
#6280=ORIENTED_EDGE('',*,*,#4922,.F.);
#6281=ORIENTED_EDGE('',*,*,#4923,.F.);
#6282=ORIENTED_EDGE('',*,*,#4924,.T.);
#6283=ORIENTED_EDGE('',*,*,#4925,.F.);
#6284=ORIENTED_EDGE('',*,*,#4920,.F.);
#6285=ORIENTED_EDGE('',*,*,#4926,.F.);
#6286=ORIENTED_EDGE('',*,*,#4927,.T.);
#6287=ORIENTED_EDGE('',*,*,#4928,.F.);
#6288=ORIENTED_EDGE('',*,*,#4924,.F.);
#6289=ORIENTED_EDGE('',*,*,#4929,.F.);
#6290=ORIENTED_EDGE('',*,*,#4930,.T.);
#6291=ORIENTED_EDGE('',*,*,#4931,.F.);
#6292=ORIENTED_EDGE('',*,*,#4927,.F.);
#6293=ORIENTED_EDGE('',*,*,#4932,.F.);
#6294=ORIENTED_EDGE('',*,*,#4933,.T.);
#6295=ORIENTED_EDGE('',*,*,#4934,.F.);
#6296=ORIENTED_EDGE('',*,*,#4930,.F.);
#6297=ORIENTED_EDGE('',*,*,#4935,.F.);
#6298=ORIENTED_EDGE('',*,*,#4936,.T.);
#6299=ORIENTED_EDGE('',*,*,#4937,.F.);
#6300=ORIENTED_EDGE('',*,*,#4933,.F.);
#6301=ORIENTED_EDGE('',*,*,#4938,.F.);
#6302=ORIENTED_EDGE('',*,*,#4939,.T.);
#6303=ORIENTED_EDGE('',*,*,#4940,.F.);
#6304=ORIENTED_EDGE('',*,*,#4936,.F.);
#6305=ORIENTED_EDGE('',*,*,#4941,.F.);
#6306=ORIENTED_EDGE('',*,*,#4942,.T.);
#6307=ORIENTED_EDGE('',*,*,#4943,.F.);
#6308=ORIENTED_EDGE('',*,*,#4939,.F.);
#6309=ORIENTED_EDGE('',*,*,#4944,.F.);
#6310=ORIENTED_EDGE('',*,*,#4945,.F.);
#6311=ORIENTED_EDGE('',*,*,#4946,.F.);
#6312=ORIENTED_EDGE('',*,*,#4942,.F.);
#6313=ORIENTED_EDGE('',*,*,#4947,.F.);
#6314=ORIENTED_EDGE('',*,*,#4948,.T.);
#6315=ORIENTED_EDGE('',*,*,#4949,.F.);
#6316=ORIENTED_EDGE('',*,*,#4950,.F.);
#6317=ORIENTED_EDGE('',*,*,#4951,.F.);
#6318=ORIENTED_EDGE('',*,*,#4952,.T.);
#6319=ORIENTED_EDGE('',*,*,#4953,.F.);
#6320=ORIENTED_EDGE('',*,*,#4948,.F.);
#6321=ORIENTED_EDGE('',*,*,#4954,.F.);
#6322=ORIENTED_EDGE('',*,*,#4955,.T.);
#6323=ORIENTED_EDGE('',*,*,#4956,.F.);
#6324=ORIENTED_EDGE('',*,*,#4952,.F.);
#6325=ORIENTED_EDGE('',*,*,#4957,.F.);
#6326=ORIENTED_EDGE('',*,*,#4958,.T.);
#6327=ORIENTED_EDGE('',*,*,#4959,.F.);
#6328=ORIENTED_EDGE('',*,*,#4955,.F.);
#6329=ORIENTED_EDGE('',*,*,#4960,.F.);
#6330=ORIENTED_EDGE('',*,*,#4961,.T.);
#6331=ORIENTED_EDGE('',*,*,#4962,.F.);
#6332=ORIENTED_EDGE('',*,*,#4958,.F.);
#6333=ORIENTED_EDGE('',*,*,#4963,.F.);
#6334=ORIENTED_EDGE('',*,*,#4964,.T.);
#6335=ORIENTED_EDGE('',*,*,#4965,.F.);
#6336=ORIENTED_EDGE('',*,*,#4961,.F.);
#6337=ORIENTED_EDGE('',*,*,#4966,.F.);
#6338=ORIENTED_EDGE('',*,*,#4967,.T.);
#6339=ORIENTED_EDGE('',*,*,#4968,.F.);
#6340=ORIENTED_EDGE('',*,*,#4964,.F.);
#6341=ORIENTED_EDGE('',*,*,#4969,.F.);
#6342=ORIENTED_EDGE('',*,*,#4970,.T.);
#6343=ORIENTED_EDGE('',*,*,#4971,.F.);
#6344=ORIENTED_EDGE('',*,*,#4967,.F.);
#6345=ORIENTED_EDGE('',*,*,#4972,.F.);
#6346=ORIENTED_EDGE('',*,*,#4973,.F.);
#6347=ORIENTED_EDGE('',*,*,#4974,.F.);
#6348=ORIENTED_EDGE('',*,*,#4970,.F.);
#6349=ORIENTED_EDGE('',*,*,#4975,.F.);
#6350=ORIENTED_EDGE('',*,*,#4976,.T.);
#6351=ORIENTED_EDGE('',*,*,#4977,.F.);
#6352=ORIENTED_EDGE('',*,*,#4976,.F.);
#6353=ORIENTED_EDGE('',*,*,#4889,.T.);
#6354=ORIENTED_EDGE('',*,*,#4978,.T.);
#6355=ORIENTED_EDGE('',*,*,#4979,.T.);
#6356=ORIENTED_EDGE('',*,*,#4980,.F.);
#6357=ORIENTED_EDGE('',*,*,#4866,.T.);
#6358=ORIENTED_EDGE('',*,*,#4981,.F.);
#6359=ORIENTED_EDGE('',*,*,#4982,.F.);
#6360=ORIENTED_EDGE('',*,*,#4983,.T.);
#6361=ORIENTED_EDGE('',*,*,#4917,.T.);
#6362=ORIENTED_EDGE('',*,*,#4984,.T.);
#6363=ORIENTED_EDGE('',*,*,#4982,.T.);
#6364=ORIENTED_EDGE('',*,*,#4985,.F.);
#6365=ORIENTED_EDGE('',*,*,#4894,.T.);
#6366=ORIENTED_EDGE('',*,*,#4986,.F.);
#6367=ORIENTED_EDGE('',*,*,#4987,.F.);
#6368=ORIENTED_EDGE('',*,*,#4988,.T.);
#6369=ORIENTED_EDGE('',*,*,#4945,.T.);
#6370=ORIENTED_EDGE('',*,*,#4989,.T.);
#6371=ORIENTED_EDGE('',*,*,#4987,.T.);
#6372=ORIENTED_EDGE('',*,*,#4990,.F.);
#6373=ORIENTED_EDGE('',*,*,#4922,.T.);
#6374=ORIENTED_EDGE('',*,*,#4991,.F.);
#6375=ORIENTED_EDGE('',*,*,#4992,.F.);
#6376=ORIENTED_EDGE('',*,*,#4993,.T.);
#6377=ORIENTED_EDGE('',*,*,#4973,.T.);
#6378=ORIENTED_EDGE('',*,*,#4994,.T.);
#6379=ORIENTED_EDGE('',*,*,#4992,.T.);
#6380=ORIENTED_EDGE('',*,*,#4995,.F.);
#6381=ORIENTED_EDGE('',*,*,#4950,.T.);
#6382=ORIENTED_EDGE('',*,*,#4996,.F.);
#6383=ORIENTED_EDGE('',*,*,#4979,.F.);
#6384=ORIENTED_EDGE('',*,*,#4997,.T.);
#6385=ORIENTED_EDGE('',*,*,#4865,.T.);
#6386=ORIENTED_EDGE('',*,*,#4869,.T.);
#6387=ORIENTED_EDGE('',*,*,#4872,.T.);
#6388=ORIENTED_EDGE('',*,*,#4875,.T.);
#6389=ORIENTED_EDGE('',*,*,#4878,.T.);
#6390=ORIENTED_EDGE('',*,*,#4881,.T.);
#6391=ORIENTED_EDGE('',*,*,#4884,.T.);
#6392=ORIENTED_EDGE('',*,*,#4887,.T.);
#6393=ORIENTED_EDGE('',*,*,#4890,.T.);
#6394=ORIENTED_EDGE('',*,*,#4980,.T.);
#6395=ORIENTED_EDGE('',*,*,#4996,.T.);
#6396=ORIENTED_EDGE('',*,*,#4949,.T.);
#6397=ORIENTED_EDGE('',*,*,#4953,.T.);
#6398=ORIENTED_EDGE('',*,*,#4956,.T.);
#6399=ORIENTED_EDGE('',*,*,#4959,.T.);
#6400=ORIENTED_EDGE('',*,*,#4962,.T.);
#6401=ORIENTED_EDGE('',*,*,#4965,.T.);
#6402=ORIENTED_EDGE('',*,*,#4968,.T.);
#6403=ORIENTED_EDGE('',*,*,#4971,.T.);
#6404=ORIENTED_EDGE('',*,*,#4974,.T.);
#6405=ORIENTED_EDGE('',*,*,#4995,.T.);
#6406=ORIENTED_EDGE('',*,*,#4991,.T.);
#6407=ORIENTED_EDGE('',*,*,#4921,.T.);
#6408=ORIENTED_EDGE('',*,*,#4925,.T.);
#6409=ORIENTED_EDGE('',*,*,#4928,.T.);
#6410=ORIENTED_EDGE('',*,*,#4931,.T.);
#6411=ORIENTED_EDGE('',*,*,#4934,.T.);
#6412=ORIENTED_EDGE('',*,*,#4937,.T.);
#6413=ORIENTED_EDGE('',*,*,#4940,.T.);
#6414=ORIENTED_EDGE('',*,*,#4943,.T.);
#6415=ORIENTED_EDGE('',*,*,#4946,.T.);
#6416=ORIENTED_EDGE('',*,*,#4990,.T.);
#6417=ORIENTED_EDGE('',*,*,#4986,.T.);
#6418=ORIENTED_EDGE('',*,*,#4893,.T.);
#6419=ORIENTED_EDGE('',*,*,#4897,.T.);
#6420=ORIENTED_EDGE('',*,*,#4900,.T.);
#6421=ORIENTED_EDGE('',*,*,#4903,.T.);
#6422=ORIENTED_EDGE('',*,*,#4906,.T.);
#6423=ORIENTED_EDGE('',*,*,#4909,.T.);
#6424=ORIENTED_EDGE('',*,*,#4912,.T.);
#6425=ORIENTED_EDGE('',*,*,#4915,.T.);
#6426=ORIENTED_EDGE('',*,*,#4918,.T.);
#6427=ORIENTED_EDGE('',*,*,#4985,.T.);
#6428=ORIENTED_EDGE('',*,*,#4981,.T.);
#6429=ORIENTED_EDGE('',*,*,#4977,.T.);
#6430=ORIENTED_EDGE('',*,*,#4863,.T.);
#6431=ORIENTED_EDGE('',*,*,#4983,.F.);
#6432=ORIENTED_EDGE('',*,*,#4984,.F.);
#6433=ORIENTED_EDGE('',*,*,#4916,.T.);
#6434=ORIENTED_EDGE('',*,*,#4913,.T.);
#6435=ORIENTED_EDGE('',*,*,#4910,.T.);
#6436=ORIENTED_EDGE('',*,*,#4907,.T.);
#6437=ORIENTED_EDGE('',*,*,#4904,.T.);
#6438=ORIENTED_EDGE('',*,*,#4901,.T.);
#6439=ORIENTED_EDGE('',*,*,#4898,.T.);
#6440=ORIENTED_EDGE('',*,*,#4895,.T.);
#6441=ORIENTED_EDGE('',*,*,#4891,.T.);
#6442=ORIENTED_EDGE('',*,*,#4988,.F.);
#6443=ORIENTED_EDGE('',*,*,#4989,.F.);
#6444=ORIENTED_EDGE('',*,*,#4944,.T.);
#6445=ORIENTED_EDGE('',*,*,#4941,.T.);
#6446=ORIENTED_EDGE('',*,*,#4938,.T.);
#6447=ORIENTED_EDGE('',*,*,#4935,.T.);
#6448=ORIENTED_EDGE('',*,*,#4932,.T.);
#6449=ORIENTED_EDGE('',*,*,#4929,.T.);
#6450=ORIENTED_EDGE('',*,*,#4926,.T.);
#6451=ORIENTED_EDGE('',*,*,#4923,.T.);
#6452=ORIENTED_EDGE('',*,*,#4919,.T.);
#6453=ORIENTED_EDGE('',*,*,#4993,.F.);
#6454=ORIENTED_EDGE('',*,*,#4994,.F.);
#6455=ORIENTED_EDGE('',*,*,#4972,.T.);
#6456=ORIENTED_EDGE('',*,*,#4969,.T.);
#6457=ORIENTED_EDGE('',*,*,#4966,.T.);
#6458=ORIENTED_EDGE('',*,*,#4963,.T.);
#6459=ORIENTED_EDGE('',*,*,#4960,.T.);
#6460=ORIENTED_EDGE('',*,*,#4957,.T.);
#6461=ORIENTED_EDGE('',*,*,#4954,.T.);
#6462=ORIENTED_EDGE('',*,*,#4951,.T.);
#6463=ORIENTED_EDGE('',*,*,#4947,.T.);
#6464=ORIENTED_EDGE('',*,*,#4997,.F.);
#6465=ORIENTED_EDGE('',*,*,#4978,.F.);
#6466=ORIENTED_EDGE('',*,*,#4888,.T.);
#6467=ORIENTED_EDGE('',*,*,#4885,.T.);
#6468=ORIENTED_EDGE('',*,*,#4882,.T.);
#6469=ORIENTED_EDGE('',*,*,#4879,.T.);
#6470=ORIENTED_EDGE('',*,*,#4876,.T.);
#6471=ORIENTED_EDGE('',*,*,#4873,.T.);
#6472=ORIENTED_EDGE('',*,*,#4870,.T.);
#6473=ORIENTED_EDGE('',*,*,#4867,.T.);
#6474=ORIENTED_EDGE('',*,*,#4975,.T.);
#7683=CYLINDRICAL_SURFACE('',#9095,0.21);
#7908=ADVANCED_FACE('',(#1236),#866,.F.);
#7909=ADVANCED_FACE('',(#1237),#867,.F.);
#7910=ADVANCED_FACE('',(#1238),#868,.F.);
#7911=ADVANCED_FACE('',(#1239),#869,.F.);
#7912=ADVANCED_FACE('',(#1240),#870,.F.);
#7913=ADVANCED_FACE('',(#1241),#871,.F.);
#7914=ADVANCED_FACE('',(#1242),#872,.F.);
#7915=ADVANCED_FACE('',(#1243),#873,.F.);
#7916=ADVANCED_FACE('',(#1244),#874,.F.);
#7917=ADVANCED_FACE('',(#1245),#875,.F.);
#7918=ADVANCED_FACE('',(#1246),#876,.F.);
#7919=ADVANCED_FACE('',(#1247),#877,.F.);
#7920=ADVANCED_FACE('',(#1248),#878,.F.);
#7921=ADVANCED_FACE('',(#1249),#879,.F.);
#7922=ADVANCED_FACE('',(#1250),#880,.F.);
#7923=ADVANCED_FACE('',(#1251),#881,.F.);
#7924=ADVANCED_FACE('',(#1252),#882,.F.);
#7925=ADVANCED_FACE('',(#1253),#883,.F.);
#7926=ADVANCED_FACE('',(#1254),#884,.F.);
#7927=ADVANCED_FACE('',(#1255),#885,.F.);
#7928=ADVANCED_FACE('',(#1256),#886,.F.);
#7929=ADVANCED_FACE('',(#1257),#887,.F.);
#7930=ADVANCED_FACE('',(#1258),#888,.F.);
#7931=ADVANCED_FACE('',(#1259),#889,.F.);
#7932=ADVANCED_FACE('',(#1260),#890,.F.);
#7933=ADVANCED_FACE('',(#1261),#891,.F.);
#7934=ADVANCED_FACE('',(#1262),#892,.F.);
#7935=ADVANCED_FACE('',(#1263),#893,.F.);
#7936=ADVANCED_FACE('',(#1264),#894,.F.);
#7937=ADVANCED_FACE('',(#1265),#895,.F.);
#7938=ADVANCED_FACE('',(#1266),#896,.F.);
#7939=ADVANCED_FACE('',(#1267),#897,.F.);
#7940=ADVANCED_FACE('',(#1268),#898,.F.);
#7941=ADVANCED_FACE('',(#1269),#899,.F.);
#7942=ADVANCED_FACE('',(#1270),#900,.F.);
#7943=ADVANCED_FACE('',(#1271),#901,.F.);
#7944=ADVANCED_FACE('',(#1272),#7683,.F.);
#7945=ADVANCED_FACE('',(#1273),#902,.T.);
#7946=ADVANCED_FACE('',(#1274),#903,.T.);
#7947=ADVANCED_FACE('',(#1275),#904,.T.);
#7948=ADVANCED_FACE('',(#1276),#905,.T.);
#7949=ADVANCED_FACE('',(#1277),#906,.T.);
#7950=ADVANCED_FACE('',(#1278),#907,.T.);
#7951=ADVANCED_FACE('',(#1279),#908,.T.);
#7952=ADVANCED_FACE('',(#1280),#909,.T.);
#7953=ADVANCED_FACE('',(#1281,#714),#910,.T.);
#7954=ADVANCED_FACE('',(#1282,#715),#911,.F.);
#8257=CLOSED_SHELL('',(#7908,#7909,#7910,#7911,#7912,#7913,#7914,#7915,
#7916,#7917,#7918,#7919,#7920,#7921,#7922,#7923,#7924,#7925,#7926,#7927,
#7928,#7929,#7930,#7931,#7932,#7933,#7934,#7935,#7936,#7937,#7938,#7939,
#7940,#7941,#7942,#7943,#7944,#7945,#7946,#7947,#7948,#7949,#7950,#7951,
#7952,#7953,#7954));
#9058=AXIS2_PLACEMENT_3D('',#13059,#10530,#10531);
#9059=AXIS2_PLACEMENT_3D('',#13060,#10532,#10533);
#9060=AXIS2_PLACEMENT_3D('',#13069,#10538,#10539);
#9061=AXIS2_PLACEMENT_3D('',#13075,#10543,#10544);
#9062=AXIS2_PLACEMENT_3D('',#13081,#10548,#10549);
#9063=AXIS2_PLACEMENT_3D('',#13087,#10553,#10554);
#9064=AXIS2_PLACEMENT_3D('',#13093,#10558,#10559);
#9065=AXIS2_PLACEMENT_3D('',#13099,#10563,#10564);
#9066=AXIS2_PLACEMENT_3D('',#13105,#10568,#10569);
#9067=AXIS2_PLACEMENT_3D('',#13111,#10573,#10574);
#9068=AXIS2_PLACEMENT_3D('',#13117,#10578,#10579);
#9069=AXIS2_PLACEMENT_3D('',#13126,#10584,#10585);
#9070=AXIS2_PLACEMENT_3D('',#13132,#10589,#10590);
#9071=AXIS2_PLACEMENT_3D('',#13138,#10594,#10595);
#9072=AXIS2_PLACEMENT_3D('',#13144,#10599,#10600);
#9073=AXIS2_PLACEMENT_3D('',#13150,#10604,#10605);
#9074=AXIS2_PLACEMENT_3D('',#13156,#10609,#10610);
#9075=AXIS2_PLACEMENT_3D('',#13162,#10614,#10615);
#9076=AXIS2_PLACEMENT_3D('',#13168,#10619,#10620);
#9077=AXIS2_PLACEMENT_3D('',#13174,#10624,#10625);
#9078=AXIS2_PLACEMENT_3D('',#13183,#10630,#10631);
#9079=AXIS2_PLACEMENT_3D('',#13189,#10635,#10636);
#9080=AXIS2_PLACEMENT_3D('',#13195,#10640,#10641);
#9081=AXIS2_PLACEMENT_3D('',#13201,#10645,#10646);
#9082=AXIS2_PLACEMENT_3D('',#13207,#10650,#10651);
#9083=AXIS2_PLACEMENT_3D('',#13213,#10655,#10656);
#9084=AXIS2_PLACEMENT_3D('',#13219,#10660,#10661);
#9085=AXIS2_PLACEMENT_3D('',#13225,#10665,#10666);
#9086=AXIS2_PLACEMENT_3D('',#13231,#10670,#10671);
#9087=AXIS2_PLACEMENT_3D('',#13240,#10676,#10677);
#9088=AXIS2_PLACEMENT_3D('',#13246,#10681,#10682);
#9089=AXIS2_PLACEMENT_3D('',#13252,#10686,#10687);
#9090=AXIS2_PLACEMENT_3D('',#13258,#10691,#10692);
#9091=AXIS2_PLACEMENT_3D('',#13264,#10696,#10697);
#9092=AXIS2_PLACEMENT_3D('',#13270,#10701,#10702);
#9093=AXIS2_PLACEMENT_3D('',#13276,#10706,#10707);
#9094=AXIS2_PLACEMENT_3D('',#13282,#10711,#10712);
#9095=AXIS2_PLACEMENT_3D('',#13288,#10716,#10717);
#9096=AXIS2_PLACEMENT_3D('',#13290,#10718,#10719);
#9097=AXIS2_PLACEMENT_3D('',#13293,#10721,#10722);
#9098=AXIS2_PLACEMENT_3D('',#13294,#10723,#10724);
#9099=AXIS2_PLACEMENT_3D('',#13300,#10728,#10729);
#9100=AXIS2_PLACEMENT_3D('',#13306,#10733,#10734);
#9101=AXIS2_PLACEMENT_3D('',#13309,#10737,#10738);
#9102=AXIS2_PLACEMENT_3D('',#13315,#10742,#10743);
#9103=AXIS2_PLACEMENT_3D('',#13318,#10746,#10747);
#9104=AXIS2_PLACEMENT_3D('',#13324,#10751,#10752);
#9105=AXIS2_PLACEMENT_3D('',#13327,#10755,#10756);
#9106=AXIS2_PLACEMENT_3D('',#13330,#10759,#10760);
#9107=AXIS2_PLACEMENT_3D('',#13331,#10761,#10762);
#10530=DIRECTION('axis',(0.,0.,1.));
#10531=DIRECTION('refdir',(1.,0.,0.));
#10532=DIRECTION('center_axis',(0.,0.,-1.));
#10533=DIRECTION('ref_axis',(0.,1.,0.));
#10534=DIRECTION('',(0.,1.,0.));
#10535=DIRECTION('',(1.,0.,0.));
#10536=DIRECTION('',(0.,-1.,0.));
#10537=DIRECTION('',(1.,0.,0.));
#10538=DIRECTION('center_axis',(0.,1.,-8.88178419700125E-16));
#10539=DIRECTION('ref_axis',(0.,8.88178419700125E-16,1.));
#10540=DIRECTION('',(0.,8.88178419700125E-16,1.));
#10541=DIRECTION('',(1.,0.,0.));
#10542=DIRECTION('',(0.,-8.88178419700125E-16,-1.));
#10543=DIRECTION('center_axis',(0.,-7.40148683083439E-16,-1.));
#10544=DIRECTION('ref_axis',(0.,1.,-7.40148683083439E-16));
#10545=DIRECTION('',(0.,1.,-7.40148683083439E-16));
#10546=DIRECTION('',(1.,0.,0.));
#10547=DIRECTION('',(0.,-1.,7.40148683083439E-16));
#10548=DIRECTION('center_axis',(0.,-0.707106781186547,-0.707106781186548));
#10549=DIRECTION('ref_axis',(0.,0.707106781186548,-0.707106781186547));
#10550=DIRECTION('',(0.,0.707106781186548,-0.707106781186547));
#10551=DIRECTION('',(1.,0.,0.));
#10552=DIRECTION('',(0.,-0.707106781186548,0.707106781186547));
#10553=DIRECTION('center_axis',(0.,-1.,2.77555756156289E-16));
#10554=DIRECTION('ref_axis',(0.,-2.77555756156289E-16,-1.));
#10555=DIRECTION('',(0.,-2.77555756156289E-16,-1.));
#10556=DIRECTION('',(1.,0.,0.));
#10557=DIRECTION('',(0.,2.77555756156289E-16,1.));
#10558=DIRECTION('center_axis',(0.,-0.707106781186547,0.707106781186548));
#10559=DIRECTION('ref_axis',(0.,-0.707106781186548,-0.707106781186547));
#10560=DIRECTION('',(0.,-0.707106781186548,-0.707106781186547));
#10561=DIRECTION('',(1.,0.,0.));
#10562=DIRECTION('',(0.,0.707106781186548,0.707106781186547));
#10563=DIRECTION('center_axis',(0.,7.40148683083438E-16,1.));
#10564=DIRECTION('ref_axis',(0.,-1.,7.40148683083438E-16));
#10565=DIRECTION('',(0.,-1.,7.40148683083438E-16));
#10566=DIRECTION('',(1.,0.,0.));
#10567=DIRECTION('',(0.,1.,-7.40148683083438E-16));
#10568=DIRECTION('center_axis',(0.,1.,-4.44089209850063E-16));
#10569=DIRECTION('ref_axis',(0.,4.44089209850063E-16,1.));
#10570=DIRECTION('',(0.,4.44089209850063E-16,1.));
#10571=DIRECTION('',(1.,0.,0.));
#10572=DIRECTION('',(0.,-4.44089209850063E-16,-1.));
#10573=DIRECTION('center_axis',(0.,2.41352831440251E-16,1.));
#10574=DIRECTION('ref_axis',(0.,-1.,2.41352831440251E-16));
#10575=DIRECTION('',(0.,-1.,2.41352831440251E-16));
#10576=DIRECTION('',(-1.,0.,0.));
#10577=DIRECTION('',(0.,1.,-2.41352831440251E-16));
#10578=DIRECTION('center_axis',(0.,-1.,2.41352831440251E-16));
#10579=DIRECTION('ref_axis',(0.,-2.41352831440251E-16,-1.));
#10580=DIRECTION('',(0.,-2.41352831440251E-16,-1.));
#10581=DIRECTION('',(1.,0.,0.));
#10582=DIRECTION('',(0.,2.41352831440251E-16,1.));
#10583=DIRECTION('',(1.,0.,0.));
#10584=DIRECTION('center_axis',(0.,0.,-1.));
#10585=DIRECTION('ref_axis',(0.,1.,0.));
#10586=DIRECTION('',(0.,1.,0.));
#10587=DIRECTION('',(1.,0.,0.));
#10588=DIRECTION('',(0.,-1.,0.));
#10589=DIRECTION('center_axis',(0.,-1.,0.));
#10590=DIRECTION('ref_axis',(0.,0.,-1.));
#10591=DIRECTION('',(0.,0.,-1.));
#10592=DIRECTION('',(1.,0.,0.));
#10593=DIRECTION('',(0.,0.,1.));
#10594=DIRECTION('center_axis',(0.,-0.707106781186547,0.707106781186548));
#10595=DIRECTION('ref_axis',(0.,-0.707106781186548,-0.707106781186547));
#10596=DIRECTION('',(0.,-0.707106781186548,-0.707106781186547));
#10597=DIRECTION('',(1.,0.,0.));
#10598=DIRECTION('',(0.,0.707106781186548,0.707106781186547));
#10599=DIRECTION('center_axis',(0.,0.,1.));
#10600=DIRECTION('ref_axis',(0.,-1.,0.));
#10601=DIRECTION('',(0.,-1.,0.));
#10602=DIRECTION('',(1.,0.,0.));
#10603=DIRECTION('',(0.,1.,0.));
#10604=DIRECTION('center_axis',(0.,0.707106781186548,0.707106781186547));
#10605=DIRECTION('ref_axis',(0.,-0.707106781186547,0.707106781186548));
#10606=DIRECTION('',(0.,-0.707106781186547,0.707106781186548));
#10607=DIRECTION('',(1.,0.,0.));
#10608=DIRECTION('',(0.,0.707106781186547,-0.707106781186548));
#10609=DIRECTION('center_axis',(0.,1.,0.));
#10610=DIRECTION('ref_axis',(0.,0.,1.));
#10611=DIRECTION('',(0.,0.,1.));
#10612=DIRECTION('',(1.,0.,0.));
#10613=DIRECTION('',(0.,0.,-1.));
#10614=DIRECTION('center_axis',(0.,0.,-1.));
#10615=DIRECTION('ref_axis',(0.,1.,0.));
#10616=DIRECTION('',(0.,1.,0.));
#10617=DIRECTION('',(1.,0.,0.));
#10618=DIRECTION('',(0.,-1.,0.));
#10619=DIRECTION('center_axis',(0.,1.,-2.41352831440251E-16));
#10620=DIRECTION('ref_axis',(0.,2.41352831440251E-16,1.));
#10621=DIRECTION('',(0.,2.41352831440251E-16,1.));
#10622=DIRECTION('',(-1.,0.,0.));
#10623=DIRECTION('',(0.,-2.41352831440251E-16,-1.));
#10624=DIRECTION('center_axis',(0.,0.,1.));
#10625=DIRECTION('ref_axis',(0.,-1.,0.));
#10626=DIRECTION('',(0.,-1.,0.));
#10627=DIRECTION('',(1.,0.,0.));
#10628=DIRECTION('',(0.,1.,0.));
#10629=DIRECTION('',(1.,0.,0.));
#10630=DIRECTION('center_axis',(0.,-1.,0.));
#10631=DIRECTION('ref_axis',(0.,0.,-1.));
#10632=DIRECTION('',(0.,0.,-1.));
#10633=DIRECTION('',(1.,0.,0.));
#10634=DIRECTION('',(0.,0.,1.));
#10635=DIRECTION('center_axis',(0.,0.,1.));
#10636=DIRECTION('ref_axis',(0.,-1.,0.));
#10637=DIRECTION('',(0.,-1.,0.));
#10638=DIRECTION('',(1.,0.,0.));
#10639=DIRECTION('',(0.,1.,0.));
#10640=DIRECTION('center_axis',(0.,0.707106781186548,0.707106781186548));
#10641=DIRECTION('ref_axis',(0.,-0.707106781186548,0.707106781186548));
#10642=DIRECTION('',(0.,-0.707106781186548,0.707106781186548));
#10643=DIRECTION('',(1.,0.,0.));
#10644=DIRECTION('',(0.,0.707106781186548,-0.707106781186548));
#10645=DIRECTION('center_axis',(0.,1.,0.));
#10646=DIRECTION('ref_axis',(0.,0.,1.));
#10647=DIRECTION('',(0.,0.,1.));
#10648=DIRECTION('',(1.,0.,0.));
#10649=DIRECTION('',(0.,0.,-1.));
#10650=DIRECTION('center_axis',(0.,0.707106781186548,-0.707106781186547));
#10651=DIRECTION('ref_axis',(0.,0.707106781186547,0.707106781186548));
#10652=DIRECTION('',(0.,0.707106781186547,0.707106781186548));
#10653=DIRECTION('',(1.,0.,0.));
#10654=DIRECTION('',(0.,-0.707106781186547,-0.707106781186548));
#10655=DIRECTION('center_axis',(0.,-7.40148683083438E-16,-1.));
#10656=DIRECTION('ref_axis',(0.,1.,-7.40148683083438E-16));
#10657=DIRECTION('',(0.,1.,-7.40148683083438E-16));
#10658=DIRECTION('',(1.,0.,0.));
#10659=DIRECTION('',(0.,-1.,7.40148683083438E-16));
#10660=DIRECTION('center_axis',(0.,-1.,0.));
#10661=DIRECTION('ref_axis',(0.,0.,-1.));
#10662=DIRECTION('',(0.,0.,-1.));
#10663=DIRECTION('',(1.,0.,0.));
#10664=DIRECTION('',(0.,0.,1.));
#10665=DIRECTION('center_axis',(0.,0.,-1.));
#10666=DIRECTION('ref_axis',(0.,1.,0.));
#10667=DIRECTION('',(0.,1.,0.));
#10668=DIRECTION('',(-1.,0.,0.));
#10669=DIRECTION('',(0.,-1.,0.));
#10670=DIRECTION('center_axis',(0.,1.,0.));
#10671=DIRECTION('ref_axis',(0.,0.,1.));
#10672=DIRECTION('',(0.,0.,1.));
#10673=DIRECTION('',(1.,0.,0.));
#10674=DIRECTION('',(0.,0.,-1.));
#10675=DIRECTION('',(1.,0.,0.));
#10676=DIRECTION('center_axis',(0.,0.,1.));
#10677=DIRECTION('ref_axis',(0.,-1.,0.));
#10678=DIRECTION('',(0.,-1.,0.));
#10679=DIRECTION('',(1.,0.,0.));
#10680=DIRECTION('',(0.,1.,0.));
#10681=DIRECTION('center_axis',(0.,1.,0.));
#10682=DIRECTION('ref_axis',(0.,0.,1.));
#10683=DIRECTION('',(0.,0.,1.));
#10684=DIRECTION('',(1.,0.,0.));
#10685=DIRECTION('',(0.,0.,-1.));
#10686=DIRECTION('center_axis',(0.,0.707106781186547,-0.707106781186548));
#10687=DIRECTION('ref_axis',(0.,0.707106781186548,0.707106781186547));
#10688=DIRECTION('',(0.,0.707106781186548,0.707106781186547));
#10689=DIRECTION('',(1.,0.,0.));
#10690=DIRECTION('',(0.,-0.707106781186548,-0.707106781186547));
#10691=DIRECTION('center_axis',(0.,0.,-1.));
#10692=DIRECTION('ref_axis',(0.,1.,0.));
#10693=DIRECTION('',(0.,1.,0.));
#10694=DIRECTION('',(1.,0.,0.));
#10695=DIRECTION('',(0.,-1.,0.));
#10696=DIRECTION('center_axis',(0.,-0.707106781186547,-0.707106781186548));
#10697=DIRECTION('ref_axis',(0.,0.707106781186548,-0.707106781186547));
#10698=DIRECTION('',(0.,0.707106781186548,-0.707106781186547));
#10699=DIRECTION('',(1.,0.,0.));
#10700=DIRECTION('',(0.,-0.707106781186548,0.707106781186547));
#10701=DIRECTION('center_axis',(0.,-1.,0.));
#10702=DIRECTION('ref_axis',(0.,0.,-1.));
#10703=DIRECTION('',(0.,0.,-1.));
#10704=DIRECTION('',(1.,0.,0.));
#10705=DIRECTION('',(0.,0.,1.));
#10706=DIRECTION('center_axis',(0.,0.,1.));
#10707=DIRECTION('ref_axis',(0.,-1.,0.));
#10708=DIRECTION('',(0.,-1.,0.));
#10709=DIRECTION('',(1.,0.,0.));
#10710=DIRECTION('',(0.,1.,0.));
#10711=DIRECTION('center_axis',(0.,-1.,0.));
#10712=DIRECTION('ref_axis',(0.,0.,-1.));
#10713=DIRECTION('',(0.,0.,-1.));
#10714=DIRECTION('',(-1.,0.,0.));
#10715=DIRECTION('',(0.,0.,1.));
#10716=DIRECTION('center_axis',(1.,0.,0.));
#10717=DIRECTION('ref_axis',(0.,0.,-1.));
#10718=DIRECTION('center_axis',(1.,0.,0.));
#10719=DIRECTION('ref_axis',(0.,0.,-1.));
#10720=DIRECTION('',(1.,0.,0.));
#10721=DIRECTION('center_axis',(-1.,0.,0.));
#10722=DIRECTION('ref_axis',(0.,0.,-1.));
#10723=DIRECTION('center_axis',(0.,1.,0.));
#10724=DIRECTION('ref_axis',(0.,0.,1.));
#10725=DIRECTION('',(0.,0.,1.));
#10726=DIRECTION('',(1.,0.,0.));
#10727=DIRECTION('',(0.,0.,1.));
#10728=DIRECTION('center_axis',(0.,1.,0.));
#10729=DIRECTION('ref_axis',(0.,0.,1.));
#10730=DIRECTION('',(0.,0.,1.));
#10731=DIRECTION('',(1.,0.,0.));
#10732=DIRECTION('',(0.,0.,1.));
#10733=DIRECTION('center_axis',(0.,0.,-1.));
#10734=DIRECTION('ref_axis',(0.,1.,0.));
#10735=DIRECTION('',(0.,1.,0.));
#10736=DIRECTION('',(0.,1.,0.));
#10737=DIRECTION('center_axis',(0.,0.,-1.));
#10738=DIRECTION('ref_axis',(0.,1.,0.));
#10739=DIRECTION('',(0.,1.,0.));
#10740=DIRECTION('',(1.,0.,0.));
#10741=DIRECTION('',(0.,1.,0.));
#10742=DIRECTION('center_axis',(0.,-1.,0.));
#10743=DIRECTION('ref_axis',(0.,0.,-1.));
#10744=DIRECTION('',(0.,0.,-1.));
#10745=DIRECTION('',(0.,0.,-1.));
#10746=DIRECTION('center_axis',(0.,-1.,0.));
#10747=DIRECTION('ref_axis',(0.,0.,-1.));
#10748=DIRECTION('',(0.,0.,-1.));
#10749=DIRECTION('',(1.,0.,0.));
#10750=DIRECTION('',(0.,0.,-1.));
#10751=DIRECTION('center_axis',(0.,0.,1.));
#10752=DIRECTION('ref_axis',(0.,-1.,0.));
#10753=DIRECTION('',(0.,-1.,0.));
#10754=DIRECTION('',(0.,-1.,0.));
#10755=DIRECTION('center_axis',(0.,0.,1.));
#10756=DIRECTION('ref_axis',(0.,-1.,0.));
#10757=DIRECTION('',(0.,-1.,0.));
#10758=DIRECTION('',(0.,-1.,0.));
#10759=DIRECTION('center_axis',(1.,0.,0.));
#10760=DIRECTION('ref_axis',(0.,0.,-1.));
#10761=DIRECTION('center_axis',(1.,0.,0.));
#10762=DIRECTION('ref_axis',(0.,0.,-1.));
#13059=CARTESIAN_POINT('',(0.,0.,0.));
#13060=CARTESIAN_POINT('Origin',(-0.1,0.82,-0.3));
#13061=CARTESIAN_POINT('',(0.,0.82,-0.3));
#13062=CARTESIAN_POINT('',(0.,1.,-0.3));
#13063=CARTESIAN_POINT('',(0.,0.41,-0.3));
#13064=CARTESIAN_POINT('',(20.,0.82,-0.3));
#13065=CARTESIAN_POINT('',(-0.1,0.82,-0.3));
#13066=CARTESIAN_POINT('',(20.,1.,-0.3));
#13067=CARTESIAN_POINT('',(20.,0.41,-0.3));
#13068=CARTESIAN_POINT('',(-0.05,1.,-0.3));
#13069=CARTESIAN_POINT('Origin',(-0.1,0.82,-0.55));
#13070=CARTESIAN_POINT('',(0.,0.82,-0.55));
#13071=CARTESIAN_POINT('',(0.,0.82,-0.275));
#13072=CARTESIAN_POINT('',(20.,0.82,-0.55));
#13073=CARTESIAN_POINT('',(-0.1,0.82,-0.55));
#13074=CARTESIAN_POINT('',(20.,0.82,-0.275));
#13075=CARTESIAN_POINT('Origin',(-0.1,0.67,-0.55));
#13076=CARTESIAN_POINT('',(0.,0.67,-0.55));
#13077=CARTESIAN_POINT('',(0.,0.335,-0.55));
#13078=CARTESIAN_POINT('',(20.,0.67,-0.55));
#13079=CARTESIAN_POINT('',(-0.1,0.67,-0.55));
#13080=CARTESIAN_POINT('',(20.,0.335,-0.55));
#13081=CARTESIAN_POINT('Origin',(-0.1,0.42,-0.3));
#13082=CARTESIAN_POINT('',(0.,0.42,-0.3));
#13083=CARTESIAN_POINT('',(0.,0.24,-0.12));
#13084=CARTESIAN_POINT('',(20.,0.42,-0.3));
#13085=CARTESIAN_POINT('',(-0.1,0.42,-0.3));
#13086=CARTESIAN_POINT('',(20.,0.24,-0.12));
#13087=CARTESIAN_POINT('Origin',(-0.1,0.42,0.3));
#13088=CARTESIAN_POINT('',(0.,0.42,0.3));
#13089=CARTESIAN_POINT('',(0.,0.42,0.15));
#13090=CARTESIAN_POINT('',(20.,0.42,0.3));
#13091=CARTESIAN_POINT('',(-0.1,0.42,0.3));
#13092=CARTESIAN_POINT('',(20.,0.42,0.15));
#13093=CARTESIAN_POINT('Origin',(-0.1,0.67,0.55));
#13094=CARTESIAN_POINT('',(0.,0.67,0.55));
#13095=CARTESIAN_POINT('',(6.93889390390723E-18,0.365,0.245));
#13096=CARTESIAN_POINT('',(20.,0.67,0.55));
#13097=CARTESIAN_POINT('',(-0.1,0.67,0.55));
#13098=CARTESIAN_POINT('',(20.,0.365,0.245));
#13099=CARTESIAN_POINT('Origin',(-0.1,0.82,0.55));
#13100=CARTESIAN_POINT('',(0.,0.82,0.55));
#13101=CARTESIAN_POINT('',(0.,0.41,0.55));
#13102=CARTESIAN_POINT('',(20.,0.82,0.55));
#13103=CARTESIAN_POINT('',(-0.1,0.82,0.55));
#13104=CARTESIAN_POINT('',(20.,0.41,0.55));
#13105=CARTESIAN_POINT('Origin',(-0.1,0.82,0.3));
#13106=CARTESIAN_POINT('',(0.,0.82,0.3));
#13107=CARTESIAN_POINT('',(0.,0.82,0.15));
#13108=CARTESIAN_POINT('',(20.,0.82,0.3));
#13109=CARTESIAN_POINT('',(-0.1,0.82,0.3));
#13110=CARTESIAN_POINT('',(20.,0.82,0.15));
#13111=CARTESIAN_POINT('Origin',(-0.1,1.05,0.3));
#13112=CARTESIAN_POINT('',(0.,1.,0.3));
#13113=CARTESIAN_POINT('',(0.,0.525,0.3));
#13114=CARTESIAN_POINT('',(20.,1.,0.3));
#13115=CARTESIAN_POINT('',(-0.05,1.,0.3));
#13116=CARTESIAN_POINT('',(20.,0.525,0.3));
#13117=CARTESIAN_POINT('Origin',(-0.1,-0.3,-0.82));
#13118=CARTESIAN_POINT('',(0.,-0.3,-0.82));
#13119=CARTESIAN_POINT('',(0.,-0.3,-1.));
#13120=CARTESIAN_POINT('',(0.,-0.3,-0.41));
#13121=CARTESIAN_POINT('',(20.,-0.3,-0.82));
#13122=CARTESIAN_POINT('',(-0.1,-0.3,-0.82));
#13123=CARTESIAN_POINT('',(20.,-0.3,-1.));
#13124=CARTESIAN_POINT('',(20.,-0.3,-0.41));
#13125=CARTESIAN_POINT('',(-0.05,-0.3,-1.));
#13126=CARTESIAN_POINT('Origin',(-0.1,-0.55,-0.82));
#13127=CARTESIAN_POINT('',(0.,-0.55,-0.82));
#13128=CARTESIAN_POINT('',(0.,-0.275,-0.82));
#13129=CARTESIAN_POINT('',(20.,-0.55,-0.82));
#13130=CARTESIAN_POINT('',(-0.1,-0.55,-0.82));
#13131=CARTESIAN_POINT('',(20.,-0.275,-0.82));
#13132=CARTESIAN_POINT('Origin',(-0.1,-0.55,-0.67));
#13133=CARTESIAN_POINT('',(0.,-0.55,-0.67));
#13134=CARTESIAN_POINT('',(0.,-0.55,-0.335));
#13135=CARTESIAN_POINT('',(20.,-0.55,-0.67));
#13136=CARTESIAN_POINT('',(-0.1,-0.55,-0.67));
#13137=CARTESIAN_POINT('',(20.,-0.55,-0.335));
#13138=CARTESIAN_POINT('Origin',(-0.1,-0.3,-0.42));
#13139=CARTESIAN_POINT('',(0.,-0.3,-0.42));
#13140=CARTESIAN_POINT('',(0.,-0.12,-0.24));
#13141=CARTESIAN_POINT('',(20.,-0.3,-0.42));
#13142=CARTESIAN_POINT('',(-0.1,-0.3,-0.42));
#13143=CARTESIAN_POINT('',(20.,-0.12,-0.24));
#13144=CARTESIAN_POINT('Origin',(-0.1,0.3,-0.42));
#13145=CARTESIAN_POINT('',(0.,0.3,-0.42));
#13146=CARTESIAN_POINT('',(0.,0.15,-0.42));
#13147=CARTESIAN_POINT('',(20.,0.3,-0.42));
#13148=CARTESIAN_POINT('',(-0.1,0.3,-0.42));
#13149=CARTESIAN_POINT('',(20.,0.15,-0.42));
#13150=CARTESIAN_POINT('Origin',(-0.1,0.55,-0.67));
#13151=CARTESIAN_POINT('',(0.,0.55,-0.67));
#13152=CARTESIAN_POINT('',(0.,0.245,-0.365));
#13153=CARTESIAN_POINT('',(20.,0.55,-0.67));
#13154=CARTESIAN_POINT('',(-0.1,0.55,-0.67));
#13155=CARTESIAN_POINT('',(20.,0.245,-0.365));
#13156=CARTESIAN_POINT('Origin',(-0.1,0.55,-0.82));
#13157=CARTESIAN_POINT('',(0.,0.55,-0.82));
#13158=CARTESIAN_POINT('',(0.,0.55,-0.41));
#13159=CARTESIAN_POINT('',(20.,0.55,-0.82));
#13160=CARTESIAN_POINT('',(-0.1,0.55,-0.82));
#13161=CARTESIAN_POINT('',(20.,0.55,-0.41));
#13162=CARTESIAN_POINT('Origin',(-0.1,0.3,-0.82));
#13163=CARTESIAN_POINT('',(0.,0.3,-0.82));
#13164=CARTESIAN_POINT('',(0.,0.15,-0.82));
#13165=CARTESIAN_POINT('',(20.,0.3,-0.82));
#13166=CARTESIAN_POINT('',(-0.1,0.3,-0.82));
#13167=CARTESIAN_POINT('',(20.,0.15,-0.82));
#13168=CARTESIAN_POINT('Origin',(-0.1,0.3,-1.05));
#13169=CARTESIAN_POINT('',(0.,0.3,-1.));
#13170=CARTESIAN_POINT('',(0.,0.3,-0.525));
#13171=CARTESIAN_POINT('',(20.,0.3,-1.));
#13172=CARTESIAN_POINT('',(-0.05,0.3,-1.));
#13173=CARTESIAN_POINT('',(20.,0.3,-0.525));
#13174=CARTESIAN_POINT('Origin',(-0.1,-0.82,0.3));
#13175=CARTESIAN_POINT('',(0.,-0.82,0.3));
#13176=CARTESIAN_POINT('',(0.,-1.,0.3));
#13177=CARTESIAN_POINT('',(0.,-0.41,0.3));
#13178=CARTESIAN_POINT('',(20.,-0.82,0.3));
#13179=CARTESIAN_POINT('',(-0.1,-0.82,0.3));
#13180=CARTESIAN_POINT('',(20.,-1.,0.3));
#13181=CARTESIAN_POINT('',(20.,-0.41,0.3));
#13182=CARTESIAN_POINT('',(-0.05,-1.,0.3));
#13183=CARTESIAN_POINT('Origin',(-0.1,-0.82,0.55));
#13184=CARTESIAN_POINT('',(0.,-0.82,0.55));
#13185=CARTESIAN_POINT('',(0.,-0.82,0.275));
#13186=CARTESIAN_POINT('',(20.,-0.82,0.55));
#13187=CARTESIAN_POINT('',(-0.1,-0.82,0.55));
#13188=CARTESIAN_POINT('',(20.,-0.82,0.275));
#13189=CARTESIAN_POINT('Origin',(-0.1,-0.67,0.55));
#13190=CARTESIAN_POINT('',(0.,-0.67,0.55));
#13191=CARTESIAN_POINT('',(0.,-0.335,0.55));
#13192=CARTESIAN_POINT('',(20.,-0.67,0.55));
#13193=CARTESIAN_POINT('',(-0.1,-0.67,0.55));
#13194=CARTESIAN_POINT('',(20.,-0.335,0.55));
#13195=CARTESIAN_POINT('Origin',(-0.1,-0.42,0.3));
#13196=CARTESIAN_POINT('',(0.,-0.42,0.3));
#13197=CARTESIAN_POINT('',(-6.93889390390723E-18,-0.24,0.12));
#13198=CARTESIAN_POINT('',(20.,-0.42,0.3));
#13199=CARTESIAN_POINT('',(-0.1,-0.42,0.3));
#13200=CARTESIAN_POINT('',(20.,-0.24,0.12));
#13201=CARTESIAN_POINT('Origin',(-0.1,-0.42,-0.3));
#13202=CARTESIAN_POINT('',(0.,-0.42,-0.3));
#13203=CARTESIAN_POINT('',(0.,-0.42,-0.15));
#13204=CARTESIAN_POINT('',(20.,-0.42,-0.3));
#13205=CARTESIAN_POINT('',(-0.1,-0.42,-0.3));
#13206=CARTESIAN_POINT('',(20.,-0.42,-0.15));
#13207=CARTESIAN_POINT('Origin',(-0.1,-0.67,-0.55));
#13208=CARTESIAN_POINT('',(0.,-0.67,-0.55));
#13209=CARTESIAN_POINT('',(0.,-0.365,-0.245));
#13210=CARTESIAN_POINT('',(20.,-0.67,-0.55));
#13211=CARTESIAN_POINT('',(-0.1,-0.67,-0.55));
#13212=CARTESIAN_POINT('',(20.,-0.365,-0.245));
#13213=CARTESIAN_POINT('Origin',(-0.1,-0.82,-0.55));
#13214=CARTESIAN_POINT('',(0.,-0.82,-0.55));
#13215=CARTESIAN_POINT('',(0.,-0.41,-0.55));
#13216=CARTESIAN_POINT('',(20.,-0.82,-0.55));
#13217=CARTESIAN_POINT('',(-0.1,-0.82,-0.55));
#13218=CARTESIAN_POINT('',(20.,-0.41,-0.55));
#13219=CARTESIAN_POINT('Origin',(-0.1,-0.82,-0.3));
#13220=CARTESIAN_POINT('',(0.,-0.82,-0.3));
#13221=CARTESIAN_POINT('',(0.,-0.82,-0.15));
#13222=CARTESIAN_POINT('',(20.,-0.82,-0.3));
#13223=CARTESIAN_POINT('',(-0.1,-0.82,-0.3));
#13224=CARTESIAN_POINT('',(20.,-0.82,-0.15));
#13225=CARTESIAN_POINT('Origin',(-0.1,-1.05,-0.3));
#13226=CARTESIAN_POINT('',(0.,-1.,-0.3));
#13227=CARTESIAN_POINT('',(0.,-0.525,-0.3));
#13228=CARTESIAN_POINT('',(20.,-1.,-0.3));
#13229=CARTESIAN_POINT('',(-0.05,-1.,-0.3));
#13230=CARTESIAN_POINT('',(20.,-0.525,-0.3));
#13231=CARTESIAN_POINT('Origin',(-0.1,0.3,0.82));
#13232=CARTESIAN_POINT('',(0.,0.3,0.82));
#13233=CARTESIAN_POINT('',(0.,0.3,1.));
#13234=CARTESIAN_POINT('',(0.,0.3,0.41));
#13235=CARTESIAN_POINT('',(20.,0.3,0.82));
#13236=CARTESIAN_POINT('',(-0.1,0.3,0.82));
#13237=CARTESIAN_POINT('',(20.,0.3,1.));
#13238=CARTESIAN_POINT('',(20.,0.3,0.41));
#13239=CARTESIAN_POINT('',(-0.05,0.3,1.));
#13240=CARTESIAN_POINT('Origin',(-0.1,0.55,0.82));
#13241=CARTESIAN_POINT('',(0.,0.55,0.82));
#13242=CARTESIAN_POINT('',(0.,0.275,0.82));
#13243=CARTESIAN_POINT('',(20.,0.55,0.82));
#13244=CARTESIAN_POINT('',(-0.1,0.55,0.82));
#13245=CARTESIAN_POINT('',(20.,0.275,0.82));
#13246=CARTESIAN_POINT('Origin',(-0.1,0.55,0.67));
#13247=CARTESIAN_POINT('',(0.,0.55,0.67));
#13248=CARTESIAN_POINT('',(0.,0.55,0.335));
#13249=CARTESIAN_POINT('',(20.,0.55,0.67));
#13250=CARTESIAN_POINT('',(-0.1,0.55,0.67));
#13251=CARTESIAN_POINT('',(20.,0.55,0.335));
#13252=CARTESIAN_POINT('Origin',(-0.1,0.3,0.42));
#13253=CARTESIAN_POINT('',(0.,0.3,0.42));
#13254=CARTESIAN_POINT('',(6.93889390390723E-18,0.12,0.24));
#13255=CARTESIAN_POINT('',(20.,0.3,0.42));
#13256=CARTESIAN_POINT('',(-0.1,0.3,0.42));
#13257=CARTESIAN_POINT('',(20.,0.12,0.24));
#13258=CARTESIAN_POINT('Origin',(-0.1,-0.3,0.42));
#13259=CARTESIAN_POINT('',(0.,-0.3,0.42));
#13260=CARTESIAN_POINT('',(0.,-0.15,0.42));
#13261=CARTESIAN_POINT('',(20.,-0.3,0.42));
#13262=CARTESIAN_POINT('',(-0.1,-0.3,0.42));
#13263=CARTESIAN_POINT('',(20.,-0.15,0.42));
#13264=CARTESIAN_POINT('Origin',(-0.1,-0.55,0.67));
#13265=CARTESIAN_POINT('',(0.,-0.55,0.67));
#13266=CARTESIAN_POINT('',(6.93889390390723E-18,-0.245,0.365));
#13267=CARTESIAN_POINT('',(20.,-0.55,0.67));
#13268=CARTESIAN_POINT('',(-0.1,-0.55,0.67));
#13269=CARTESIAN_POINT('',(20.,-0.245,0.365));
#13270=CARTESIAN_POINT('Origin',(-0.1,-0.55,0.82));
#13271=CARTESIAN_POINT('',(0.,-0.55,0.82));
#13272=CARTESIAN_POINT('',(0.,-0.55,0.41));
#13273=CARTESIAN_POINT('',(20.,-0.55,0.82));
#13274=CARTESIAN_POINT('',(-0.1,-0.55,0.82));
#13275=CARTESIAN_POINT('',(20.,-0.55,0.41));
#13276=CARTESIAN_POINT('Origin',(-0.1,-0.3,0.82));
#13277=CARTESIAN_POINT('',(0.,-0.3,0.82));
#13278=CARTESIAN_POINT('',(0.,-0.15,0.82));
#13279=CARTESIAN_POINT('',(20.,-0.3,0.82));
#13280=CARTESIAN_POINT('',(-0.1,-0.3,0.82));
#13281=CARTESIAN_POINT('',(20.,-0.15,0.82));
#13282=CARTESIAN_POINT('Origin',(-0.1,-0.3,1.05));
#13283=CARTESIAN_POINT('',(0.,-0.3,1.));
#13284=CARTESIAN_POINT('',(0.,-0.3,0.525));
#13285=CARTESIAN_POINT('',(20.,-0.3,1.));
#13286=CARTESIAN_POINT('',(-0.05,-0.3,1.));
#13287=CARTESIAN_POINT('',(20.,-0.3,0.525));
#13288=CARTESIAN_POINT('Origin',(-0.1,0.,0.));
#13289=CARTESIAN_POINT('',(0.,-2.57175827820944E-17,0.21));
#13290=CARTESIAN_POINT('Origin',(0.,0.,0.));
#13291=CARTESIAN_POINT('',(20.,2.57175827820944E-17,0.21));
#13292=CARTESIAN_POINT('',(-0.1,-2.57175827820944E-17,0.21));
#13293=CARTESIAN_POINT('Origin',(20.,0.,0.));
#13294=CARTESIAN_POINT('Origin',(0.,1.,-1.));
#13295=CARTESIAN_POINT('',(0.,1.,1.));
#13296=CARTESIAN_POINT('',(0.,1.,-1.));
#13297=CARTESIAN_POINT('',(20.,1.,1.));
#13298=CARTESIAN_POINT('',(0.,1.,1.));
#13299=CARTESIAN_POINT('',(20.,1.,-1.));
#13300=CARTESIAN_POINT('Origin',(0.,1.,-1.));
#13301=CARTESIAN_POINT('',(20.,1.,-1.));
#13302=CARTESIAN_POINT('',(20.,1.,-1.));
#13303=CARTESIAN_POINT('',(0.,1.,-1.));
#13304=CARTESIAN_POINT('',(0.,1.,-1.));
#13305=CARTESIAN_POINT('',(0.,1.,-1.));
#13306=CARTESIAN_POINT('Origin',(0.,-1.,-1.));
#13307=CARTESIAN_POINT('',(0.,-1.,-1.));
#13308=CARTESIAN_POINT('',(20.,-1.,-1.));
#13309=CARTESIAN_POINT('Origin',(0.,-1.,-1.));
#13310=CARTESIAN_POINT('',(20.,-1.,-1.));
#13311=CARTESIAN_POINT('',(20.,-1.,-1.));
#13312=CARTESIAN_POINT('',(0.,-1.,-1.));
#13313=CARTESIAN_POINT('',(0.,-1.,-1.));
#13314=CARTESIAN_POINT('',(0.,-1.,-1.));
#13315=CARTESIAN_POINT('Origin',(0.,-1.,1.));
#13316=CARTESIAN_POINT('',(0.,-1.,1.));
#13317=CARTESIAN_POINT('',(20.,-1.,1.));
#13318=CARTESIAN_POINT('Origin',(0.,-1.,1.));
#13319=CARTESIAN_POINT('',(20.,-1.,1.));
#13320=CARTESIAN_POINT('',(20.,-1.,1.));
#13321=CARTESIAN_POINT('',(0.,-1.,1.));
#13322=CARTESIAN_POINT('',(0.,-1.,1.));
#13323=CARTESIAN_POINT('',(0.,-1.,1.));
#13324=CARTESIAN_POINT('Origin',(0.,1.,1.));
#13325=CARTESIAN_POINT('',(0.,1.,1.));
#13326=CARTESIAN_POINT('',(20.,1.,1.));
#13327=CARTESIAN_POINT('Origin',(0.,1.,1.));
#13328=CARTESIAN_POINT('',(20.,1.,1.));
#13329=CARTESIAN_POINT('',(0.,1.,1.));
#13330=CARTESIAN_POINT('Origin',(20.,0.,0.));
#13331=CARTESIAN_POINT('Origin',(0.,0.,0.));
#15127=UNCERTAINTY_MEASURE_WITH_UNIT(LENGTH_MEASURE(0.001),#15213,
'DISTANCE_ACCURACY_VALUE',
'Maximum model space distance between geometric entities at asserted c
onnectivities');
#15162=UNCERTAINTY_MEASURE_WITH_UNIT(LENGTH_MEASURE(0.001),#15213,
'DISTANCE_ACCURACY_VALUE',
'Maximum model space distance between geometric entities at asserted c
onnectivities');
#15177=(
GEOMETRIC_REPRESENTATION_CONTEXT(3)
GLOBAL_UNCERTAINTY_ASSIGNED_CONTEXT((#15127))
GLOBAL_UNIT_ASSIGNED_CONTEXT((#15213,#15215,#15216))
REPRESENTATION_CONTEXT('','3D')
);
#15212=(
GEOMETRIC_REPRESENTATION_CONTEXT(3)
GLOBAL_UNCERTAINTY_ASSIGNED_CONTEXT((#15162))
GLOBAL_UNIT_ASSIGNED_CONTEXT((#15213,#15215,#15216))
REPRESENTATION_CONTEXT('','3D')
);
#15213=(
LENGTH_UNIT()
NAMED_UNIT(*)
SI_UNIT(.CENTI.,.METRE.)
);
#15215=(
NAMED_UNIT(*)
PLANE_ANGLE_UNIT()
SI_UNIT($,.RADIAN.)
);
#15216=(
NAMED_UNIT(*)
SI_UNIT($,.STERADIAN.)
SOLID_ANGLE_UNIT()
);
#15231=SHAPE_DEFINITION_REPRESENTATION(#15280,#15415);
#15280=PRODUCT_DEFINITION_SHAPE('',$,#15465);
#15415=SHAPE_REPRESENTATION('',(#9058),#15177);
#15450=PRODUCT_DEFINITION_CONTEXT('part definition',#15599,'design');
#15465=PRODUCT_DEFINITION('Slotted Extrusion - 20 x 20 x 200 mm',
'Slotted Extrusion - 20 x 20 x 200 mm',#15514,#15450);
#15514=PRODUCT_DEFINITION_FORMATION('',$,#15615);
#15599=APPLICATION_CONTEXT(
'Core Data for Automotive Mechanical Design Process');
#15600=PRODUCT_CONTEXT('part definition',#15599,'mechanical');
#15615=PRODUCT('Slotted Extrusion - 20 x 20 x 200 mm',
'Slotted Extrusion - 20 x 20 x 200 mm',
'Slotted Extrusion - 20 x 20 x 200 mm',(#15600));
#15727=COLOUR_RGB('Off White',0.89,0.88,0.83);
#15728=FILL_AREA_STYLE_COLOUR('',#15727);
#15729=FILL_AREA_STYLE('',(#15728));
#15730=SURFACE_STYLE_FILL_AREA(#15729);
#15731=SURFACE_SIDE_STYLE('',(#15730));
#15732=SURFACE_STYLE_USAGE(.BOTH.,#15731);
#15733=PRESENTATION_STYLE_ASSIGNMENT((#15732));
ENDSEC;
END-ISO-10303-21;
